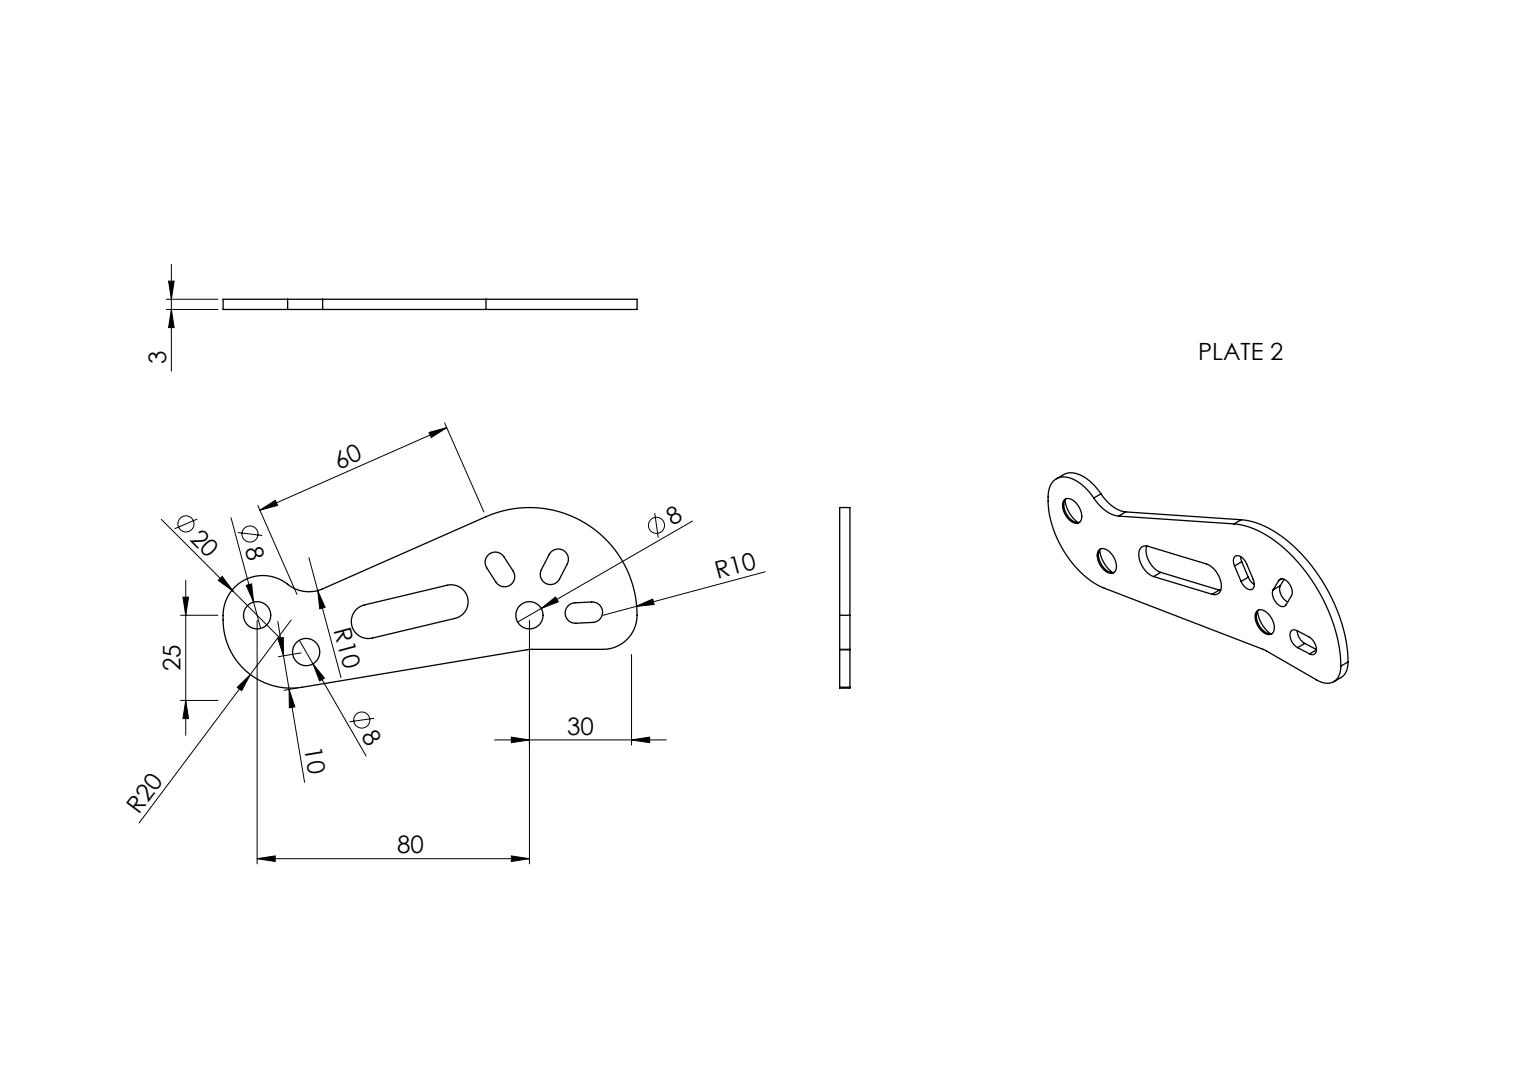
ISO-10303-21;
HEADER;
FILE_DESCRIPTION (('STEP AP214'),
    '1' );
FILE_NAME ('plate 2.step',
    '2026-10-31T03:41:51',
    ( '' ),
    ( '' ),
    'SwSTEP 2.0',
    'SolidWorks 2026',
    '' );
FILE_SCHEMA (( 'AUTOMOTIVE_DESIGN' ));
ENDSEC;

DATA;
#18=ORIENTED_EDGE ( 'NONE', *, *, #2231, .T. ) ;
#36=ORIENTED_EDGE ( 'NONE', *, *, #1393, .T. ) ;
#45=FACE_OUTER_BOUND ( 'NONE', #11478, .T. ) ;
#51=CARTESIAN_POINT ( 'NONE',  ( 69.97572749000833880, 15.55805301486455683, 6.000000000000000000 ) ) ;
#52=ORIENTED_EDGE ( 'NONE', *, *, #8148, .F. ) ;
#97=ADVANCED_FACE ( 'NONE', ( #2039 ), #6726, .F. ) ;
#108=VERTEX_POINT ( 'NONE', #10337 ) ;
#117=CARTESIAN_POINT ( 'NONE',  ( 76.00000000000000000, 4.898587196589422689E-16, 6.000000000000000000 ) ) ;
#123=EDGE_LOOP ( 'NONE', ( #11142, #6694, #3229, #3331, #1477 ) ) ;
#135=CARTESIAN_POINT ( 'NONE',  ( 80.00000000000000000, 0.000000000000000000, 5.500000000000000000 ) ) ;
#145=VECTOR ( 'NONE', #5198, 1000.000000000000000 ) ;
#158=DIRECTION ( 'NONE',  ( 1.000000000000000000, 0.000000000000000000, 0.000000000000000000 ) ) ;
#160=VECTOR ( 'NONE', #9182, 1000.000000000000000 ) ;
#161=LINE ( 'NONE', #4805, #11382 ) ;
#186=PLANE ( 'NONE',  #13689 ) ;
#193=ORIENTED_EDGE ( 'NONE', *, *, #9161, .T. ) ;
#211=EDGE_CURVE ( 'NONE', #12769, #12700, #14657, .T. ) ;
#214=VERTEX_POINT ( 'NONE', #2422 ) ;
#216=CARTESIAN_POINT ( 'NONE',  ( 80.00000000000000000, 0.000000000000000000, -131.1575142076926852 ) ) ;
#224=DIRECTION ( 'NONE',  ( -0.000000000000000000, -0.000000000000000000, -1.000000000000000000 ) ) ;
#233=DIRECTION ( 'NONE',  ( 1.000000000000000000, 0.000000000000000000, 0.000000000000000000 ) ) ;
#234=ADVANCED_FACE ( 'NONE', ( #9266 ), #13953, .F. ) ;
#239=DIRECTION ( 'NONE',  ( 0.9728364810787194505, 0.2314933715733012709, -0.000000000000000000 ) ) ;
#243=CARTESIAN_POINT ( 'NONE',  ( 31.51081190520435626, 3.030430839836910639, 2.999999999999999112 ) ) ;
#244=LINE ( 'NONE', #4960, #10717 ) ;
#246=CARTESIAN_POINT ( 'NONE',  ( 10.40394475573011945, -10.79473832354794460, 6.000000000000000000 ) ) ;
#247=ORIENTED_EDGE ( 'NONE', *, *, #4486, .T. ) ;
#250=CARTESIAN_POINT ( 'NONE',  ( -5.999999999999999112, 0.000000000000000000, 3.000000000000000000 ) ) ;
#253=( LENGTH_UNIT ( ) NAMED_UNIT ( * ) SI_UNIT ( .MILLI., .METRE. ) );
#264=EDGE_CURVE ( 'NONE', #12037, #12700, #1561, .T. ) ;
#289=DIRECTION ( 'NONE',  ( 1.000000000000000000, 0.000000000000000000, -0.000000000000000000 ) ) ;
#310=FACE_OUTER_BOUND ( 'NONE', #10572, .T. ) ;
#314=DIRECTION ( 'NONE',  ( -0.000000000000000000, -0.000000000000000000, -1.000000000000000000 ) ) ;
#326=DIRECTION ( 'NONE',  ( 0.000000000000000000, 0.000000000000000000, 1.000000000000000000 ) ) ;
#332=DIRECTION ( 'NONE',  ( 1.000000000000000000, 0.000000000000000000, 0.000000000000000000 ) ) ;
#340=EDGE_CURVE ( 'NONE', #7818, #11509, #2563, .T. ) ;
#344=EDGE_CURVE ( 'NONE', #1013, #13731, #244, .T. ) ;
#351=DIRECTION ( 'NONE',  ( -0.000000000000000000, -0.000000000000000000, -1.000000000000000000 ) ) ;
#372=DIRECTION ( 'NONE',  ( -0.000000000000000000, -0.000000000000000000, 1.000000000000000000 ) ) ;
#401=AXIS2_PLACEMENT_3D ( 'NONE', #216, #3759, #10608 ) ;
#412=LINE ( 'NONE', #6346, #4643 ) ;
#413=DIRECTION ( 'NONE',  ( -0.000000000000000000, -0.000000000000000000, 1.000000000000000000 ) ) ;
#445=CARTESIAN_POINT ( 'NONE',  ( 19.25177984293775424, 7.759396820770413150, 6.000000000000005329 ) ) ;
#454=DIRECTION ( 'NONE',  ( -1.000000000000000000, 0.000000000000000000, 0.000000000000000000 ) ) ;
#460=EDGE_CURVE ( 'NONE', #5313, #7859, #6354, .T. ) ;
#466=ORIENTED_EDGE ( 'NONE', *, *, #12652, .F. ) ;
#470=ORIENTED_EDGE ( 'NONE', *, *, #13886, .T. ) ;
#480=CARTESIAN_POINT ( 'NONE',  ( -9.999999999999998224, 0.000000000000000000, -131.1575142076926852 ) ) ;
#481=ORIENTED_EDGE ( 'NONE', *, *, #1964, .T. ) ;
#487=CYLINDRICAL_SURFACE ( 'NONE', #11244, 5.999999999999999112 ) ;
#491=CARTESIAN_POINT ( 'NONE',  ( 67.23404255319148604, 28.93147646537027384, -131.1575142076926852 ) ) ;
#501=DIRECTION ( 'NONE',  ( -1.000000000000000000, 0.000000000000000000, 0.000000000000000000 ) ) ;
#511=EDGE_CURVE ( 'NONE', #12603, #7404, #14471, .T. ) ;
#518=CARTESIAN_POINT ( 'NONE',  ( 80.00000000000000000, 0.000000000000000000, -131.1575142076926852 ) ) ;
#534=VECTOR ( 'NONE', #1828, 1000.000000000000000 ) ;
#538=CARTESIAN_POINT ( 'NONE',  ( 69.97572749000833880, 15.55805301486455683, 2.999999999999999112 ) ) ;
#541=ORIENTED_EDGE ( 'NONE', *, *, #8159, .F. ) ;
#548=LINE ( 'NONE', #11154, #9933 ) ;
#550=LINE ( 'NONE', #5266, #14058 ) ;
#554=CARTESIAN_POINT ( 'NONE',  ( 31.51081190520435626, 3.030430839836910639, 2.999999999999999112 ) ) ;
#555=VERTEX_POINT ( 'NONE', #13184 ) ;
#558=FILL_AREA_STYLE ('',( #14571 ) ) ;
#562=ORIENTED_EDGE ( 'NONE', *, *, #11530, .T. ) ;
#578=VECTOR ( 'NONE', #11844, 1000.000000000000000 ) ;
#596=ORIENTED_EDGE ( 'NONE', *, *, #3350, .T. ) ;
#605=VECTOR ( 'NONE', #5620, 1000.000000000000114 ) ;
#614=AXIS2_PLACEMENT_3D ( 'NONE', #11477, #5656, #729 ) ;
#664=DIRECTION ( 'NONE',  ( 0.000000000000000000, 0.000000000000000000, 1.000000000000000000 ) ) ;
#666=PRODUCT_CONTEXT ( 'NONE', #2624, 'mechanical' ) ;
#677=VERTEX_POINT ( 'NONE', #4761 ) ;
#679=DIRECTION ( 'NONE',  ( 1.000000000000000000, 0.000000000000000000, 0.000000000000000000 ) ) ;
#682=ORIENTED_EDGE ( 'NONE', *, *, #8049, .T. ) ;
#708=AXIS2_PLACEMENT_3D ( 'NONE', #5305, #9976, #14676 ) ;
#714=LINE ( 'NONE', #863, #6086 ) ;
#729=DIRECTION ( 'NONE',  ( 1.000000000000000000, 0.000000000000000000, 0.000000000000000000 ) ) ;
#746=ADVANCED_FACE ( 'NONE', ( #2228 ), #6914, .F. ) ;
#747=CARTESIAN_POINT ( 'NONE',  ( -4.000000000000000000, 0.000000000000000000, 6.000000000000000000 ) ) ;
#779=EDGE_CURVE ( 'NONE', #11305, #1805, #11744, .T. ) ;
#788=ORIENTED_EDGE ( 'NONE', *, *, #5470, .F. ) ;
#794=AXIS2_PLACEMENT_3D ( 'NONE', #9301, #8135, #991 ) ;
#854=AXIS2_PLACEMENT_3D ( 'NONE', #10836, #10689, #6078 ) ;
#855=AXIS2_PLACEMENT_3D ( 'NONE', #5788, #13776, #8092 ) ;
#861=DIRECTION ( 'NONE',  ( 0.000000000000000000, 0.000000000000000000, 1.000000000000000000 ) ) ;
#862=FACE_OUTER_BOUND ( 'NONE', #14868, .T. ) ;
#863=CARTESIAN_POINT ( 'NONE',  ( 31.51081190520435626, 3.030430839836910639, 2.999999999999999112 ) ) ;
#864=AXIS2_PLACEMENT_3D ( 'NONE', #2501, #3652, #7037 ) ;
#870=ORIENTED_EDGE ( 'NONE', *, *, #10742, .T. ) ;
#877=ORIENTED_EDGE ( 'NONE', *, *, #7016, .T. ) ;
#878=CARTESIAN_POINT ( 'NONE',  ( -9.999999999999998224, 0.000000000000000000, -131.1575142076926852 ) ) ;
#904=EDGE_LOOP ( 'NONE', ( #11080, #1437, #4193, #4487 ) ) ;
#913=LINE ( 'NONE', #4463, #605 ) ;
#926=AXIS2_PLACEMENT_3D ( 'NONE', #8242, #7946, #12629 ) ;
#937=CIRCLE ( 'NONE', #9527, 4.000000000000003553 ) ;
#961=( LENGTH_UNIT ( ) NAMED_UNIT ( * ) SI_UNIT ( .MILLI., .METRE. ) );
#976=DIRECTION ( 'NONE',  ( -1.000000000000000000, 0.000000000000000000, 0.000000000000000000 ) ) ;
#977=VECTOR ( 'NONE', #5224, 1000.000000000000000 ) ;
#979=ORIENTED_EDGE ( 'NONE', *, *, #5847, .F. ) ;
#981=CARTESIAN_POINT ( 'NONE',  ( 15.21482963846748504, 16.90833299098317610, 3.000000000000002665 ) ) ;
#991=DIRECTION ( 'NONE',  ( -1.000000000000000000, 0.000000000000000000, -0.000000000000000000 ) ) ;
#994=DIRECTION ( 'NONE',  ( 1.000000000000000000, 0.000000000000000000, 0.000000000000000000 ) ) ;
#1013=VERTEX_POINT ( 'NONE', #13943 ) ;
#1041=ORIENTED_EDGE ( 'NONE', *, *, #264, .T. ) ;
#1044=EDGE_CURVE ( 'NONE', #5009, #9526, #161, .T. ) ;
#1059=DIRECTION ( 'NONE',  ( -0.000000000000000000, -0.000000000000000000, 1.000000000000000000 ) ) ;
#1075=EDGE_LOOP ( 'NONE', ( #12142, #6161 ) ) ;
#1078=ORIENTED_EDGE ( 'NONE', *, *, #5790, .F. ) ;
#1079=EDGE_LOOP ( 'NONE', ( #2513, #15023, #6182, #877 ) ) ;
#1098=ORIENTED_EDGE ( 'NONE', *, *, #9625, .T. ) ;
#1109=LINE ( 'NONE', #4729, #8437 ) ;
#1114=CIRCLE ( 'NONE', #5058, 2.999999999999975131 ) ;
#1136=VERTEX_POINT ( 'NONE', #10785 ) ;
#1161=PLANE ( 'NONE',  #7041 ) ;
#1163=( GEOMETRIC_REPRESENTATION_CONTEXT ( 3 ) GLOBAL_UNCERTAINTY_ASSIGNED_CONTEXT ( ( #8003 ) ) GLOBAL_UNIT_ASSIGNED_CONTEXT ( ( #961, #13644, #10039 ) ) REPRESENTATION_CONTEXT ( 'NONE', 'WORKASPACE' ) );
#1174=CARTESIAN_POINT ( 'NONE',  ( 8.961831343790189308, 9.104486995144789319, 3.000000000000002665 ) ) ;
#1185=CARTESIAN_POINT ( 'NONE',  ( 83.50748565343083385, 13.38500995229612478, 2.999999999999999112 ) ) ;
#1218=DIRECTION ( 'NONE',  ( 0.000000000000000000, 0.000000000000000000, -1.000000000000000000 ) ) ;
#1225=DIRECTION ( 'NONE',  ( 0.2314933715733012709, -0.9728364810787194505, 0.000000000000000000 ) ) ;
#1236=CYLINDRICAL_SURFACE ( 'NONE', #401, 31.62277660168379256 ) ;
#1247=EDGE_CURVE ( 'NONE', #7097, #4081, #548, .T. ) ;
#1250=CARTESIAN_POINT ( 'NONE',  ( 10.40394475573011945, -10.79473832354794460, 6.000000000000000000 ) ) ;
#1253=LINE ( 'NONE', #10562, #4367 ) ;
#1280=LINE ( 'NONE', #8132, #6582 ) ;
#1287=ORIENTED_EDGE ( 'NONE', *, *, #1044, .T. ) ;
#1297=ORIENTED_EDGE ( 'NONE', *, *, #12952, .T. ) ;
#1300=FACE_OUTER_BOUND ( 'NONE', #5332, .T. ) ;
#1346=CARTESIAN_POINT ( 'NONE',  ( 18.40394475573011945, -10.79473832354794460, 6.000000000000000000 ) ) ;
#1361=LINE ( 'NONE', #2683, #9152 ) ;
#1364=ORIENTED_EDGE ( 'NONE', *, *, #11141, .T. ) ;
#1369=CARTESIAN_POINT ( 'NONE',  ( 0.000000000000000000, 0.000000000000000000, 5.500000000000000000 ) ) ;
#1376=AXIS2_PLACEMENT_3D ( 'NONE', #7353, #6187, #9640 ) ;
#1382=DIRECTION ( 'NONE',  ( -0.000000000000000000, -0.000000000000000000, 1.000000000000000000 ) ) ;
#1384=EDGE_CURVE ( 'NONE', #1805, #14461, #7483, .T. ) ;
#1392=AXIS2_PLACEMENT_3D ( 'NONE', #12930, #7026, #11705 ) ;
#1393=EDGE_CURVE ( 'NONE', #11633, #7557, #3313, .T. ) ;
#1407=ADVANCED_FACE ( 'NONE', ( #862 ), #10161, .F. ) ;
#1411=CARTESIAN_POINT ( 'NONE',  ( 80.00000000000000000, 0.000000000000000000, 3.000000000000002665 ) ) ;
#1419=AXIS2_PLACEMENT_3D ( 'NONE', #9521, #10244, #11889 ) ;
#1425=LINE ( 'NONE', #5277, #6096 ) ;
#1429=AXIS2_PLACEMENT_3D ( 'NONE', #14450, #12280, #8594 ) ;
#1437=ORIENTED_EDGE ( 'NONE', *, *, #3878, .F. ) ;
#1453=CARTESIAN_POINT ( 'NONE',  ( 74.00000000000000000, 0.000000000000000000, 5.500000000000000000 ) ) ;
#1469=CARTESIAN_POINT ( 'NONE',  ( 80.00000000000000000, -9.999999999999994671, -131.1575142076926852 ) ) ;
#1470=DIRECTION ( 'NONE',  ( 0.000000000000000000, 0.000000000000000000, -1.000000000000000000 ) ) ;
#1477=ORIENTED_EDGE ( 'NONE', *, *, #1540, .F. ) ;
#1482=VERTEX_POINT ( 'NONE', #8309 ) ;
#1494=ORIENTED_EDGE ( 'NONE', *, *, #4486, .F. ) ;
#1502=DIRECTION ( 'NONE',  ( 0.000000000000000000, 0.000000000000000000, 1.000000000000000000 ) ) ;
#1518=DIRECTION ( 'NONE',  ( -0.000000000000000000, -0.000000000000000000, 1.000000000000000000 ) ) ;
#1523=DIRECTION ( 'NONE',  ( 1.000000000000000000, 0.000000000000000000, 0.000000000000000000 ) ) ;
#1524=VECTOR ( 'NONE', #2212, 1000.000000000000000 ) ;
#1526=DIRECTION ( 'NONE',  ( 0.000000000000000000, 0.000000000000000000, 1.000000000000000000 ) ) ;
#1527=EDGE_CURVE ( 'NONE', #14446, #9599, #1641, .T. ) ;
#1532=EDGE_LOOP ( 'NONE', ( #3117, #4460, #13209, #9461, #14696 ) ) ;
#1539=CARTESIAN_POINT ( 'NONE',  ( 10.00000000000000178, -1.390791565672601315, 3.000000000000002665 ) ) ;
#1540=EDGE_CURVE ( 'NONE', #14414, #5535, #6005, .T. ) ;
#1551=EDGE_LOOP ( 'NONE', ( #3528, #541, #2755, #9080, #10467 ) ) ;
#1559=ORIENTED_EDGE ( 'NONE', *, *, #5818, .T. ) ;
#1560=DIRECTION ( 'NONE',  ( 1.000000000000000000, 0.000000000000000000, 0.000000000000000000 ) ) ;
#1561=LINE ( 'NONE', #480, #145 ) ;
#1570=EDGE_CURVE ( 'NONE', #2216, #4678, #12832, .T. ) ;
#1571=EDGE_CURVE ( 'NONE', #13989, #10279, #3470, .T. ) ;
#1589=VECTOR ( 'NONE', #7529, 1000.000000000000000 ) ;
#1603=EDGE_CURVE ( 'NONE', #1860, #1482, #7085, .T. ) ;
#1641=CIRCLE ( 'NONE', #6308, 4.999999999999997335 ) ;
#1643=DIRECTION ( 'NONE',  ( 0.04874958797097354163, -0.9988110320138942066, 0.000000000000000000 ) ) ;
#1655=( NAMED_UNIT ( * ) SI_UNIT ( $, .STERADIAN. ) SOLID_ANGLE_UNIT ( ) );
#1659=ORIENTED_EDGE ( 'NONE', *, *, #4604, .F. ) ;
#1669=ORIENTED_EDGE ( 'NONE', *, *, #460, .T. ) ;
#1671=VECTOR ( 'NONE', #11024, 1000.000000000000000 ) ;
#1675=VECTOR ( 'NONE', #9164, 1000.000000000000227 ) ;
#1682=ORIENTED_EDGE ( 'NONE', *, *, #11497, .T. ) ;
#1685=CARTESIAN_POINT ( 'NONE',  ( 85.79342132543153809, 17.83186255874426962, 6.000000000000000000 ) ) ;
#1693=ORIENTED_EDGE ( 'NONE', *, *, #9686, .T. ) ;
#1703=LINE ( 'NONE', #8538, #10944 ) ;
#1704=DIRECTION ( 'NONE',  ( 1.000000000000000000, 0.000000000000000000, 0.000000000000000000 ) ) ;
#1706=ORIENTED_EDGE ( 'NONE', *, *, #3827, .F. ) ;
#1719=VECTOR ( 'NONE', #8136, 1000.000000000000000 ) ;
#1725=CARTESIAN_POINT ( 'NONE',  ( 56.98919079003883326, 3.953582723775848962, 2.999999999999999112 ) ) ;
#1732=EDGE_CURVE ( 'NONE', #3235, #9526, #15133, .T. ) ;
#1734=EDGE_CURVE ( 'NONE', #14461, #2630, #1703, .T. ) ;
#1769=EDGE_CURVE ( 'NONE', #13658, #11133, #8990, .T. ) ;
#1776=CIRCLE ( 'NONE', #6200, 5.999999999999999112 ) ;
#1788=EDGE_LOOP ( 'NONE', ( #2878, #682, #5226, #13096 ) ) ;
#1800=CARTESIAN_POINT ( 'NONE',  ( -9.999999999999992895, -25.00000000000000000, -131.1575142076926852 ) ) ;
#1803=DIRECTION ( 'NONE',  ( 0.000000000000000000, 0.000000000000000000, 1.000000000000000000 ) ) ;
#1805=VERTEX_POINT ( 'NONE', #5475 ) ;
#1808=ORIENTED_EDGE ( 'NONE', *, *, #6015, .T. ) ;
#1828=DIRECTION ( 'NONE',  ( -0.000000000000000000, -0.000000000000000000, -1.000000000000000000 ) ) ;
#1830=DIRECTION ( 'NONE',  ( 1.000000000000000000, 0.000000000000000000, 0.000000000000000000 ) ) ;
#1860=VERTEX_POINT ( 'NONE', #11521 ) ;
#1865=CYLINDRICAL_SURFACE ( 'NONE', #10935, 2.999999999999988898 ) ;
#1874=AXIS2_PLACEMENT_3D ( 'NONE', #1369, #10753, #11665 ) ;
#1895=CARTESIAN_POINT ( 'NONE',  ( 76.00000000000000000, 4.898587196589422689E-16, 5.500000000000005329 ) ) ;
#1905=CARTESIAN_POINT ( 'NONE',  ( 0.000000000000000000, 0.000000000000000000, 5.500000000000000000 ) ) ;
#1913=ORIENTED_EDGE ( 'NONE', *, *, #9541, .F. ) ;
#1915=STYLED_ITEM ( 'NONE', ( #6714 ), #15172 ) ;
#1921=AXIS2_PLACEMENT_3D ( 'NONE', #4330, #13703, #3182 ) ;
#1925=DIRECTION ( 'NONE',  ( 0.000000000000000000, 0.000000000000000000, 1.000000000000000000 ) ) ;
#1929=DIRECTION ( 'NONE',  ( -1.000000000000000000, 0.000000000000000000, 0.000000000000000000 ) ) ;
#1946=AXIS2_PLACEMENT_3D ( 'NONE', #3215, #10121, #11276 ) ;
#1947=CARTESIAN_POINT ( 'NONE',  ( 70.16198417812034904, 9.730076655429538590, 2.999999999999999112 ) ) ;
#1964=EDGE_CURVE ( 'NONE', #4081, #10279, #8485, .T. ) ;
#1976=ORIENTED_EDGE ( 'NONE', *, *, #6296, .T. ) ;
#1981=ADVANCED_FACE ( 'NONE', ( #5985 ), #3522, .F. ) ;
#1992=ADVANCED_FACE ( 'NONE', ( #8139 ), #6987, .F. ) ;
#2001=CARTESIAN_POINT ( 'NONE',  ( 101.6227766016837819, 5.204170427930421283E-15, -131.1575142076926852 ) ) ;
#2020=LINE ( 'NONE', #13546, #4525 ) ;
#2029=SURFACE_STYLE_FILL_AREA ( #558 ) ;
#2033=DIRECTION ( 'NONE',  ( 1.000000000000000000, 0.000000000000000000, 0.000000000000000000 ) ) ;
#2039=FACE_OUTER_BOUND ( 'NONE', #8512, .T. ) ;
#2044=DIRECTION ( 'NONE',  ( -0.000000000000000000, -0.000000000000000000, 1.000000000000000000 ) ) ;
#2060=DIRECTION ( 'NONE',  ( 0.000000000000000000, 0.000000000000000000, 1.000000000000000000 ) ) ;
#2062=ORIENTED_EDGE ( 'NONE', *, *, #1527, .F. ) ;
#2086=FACE_OUTER_BOUND ( 'NONE', #13410, .T. ) ;
#2109=CARTESIAN_POINT ( 'NONE',  ( 0.000000000000000000, 0.000000000000000000, 3.000000000000000000 ) ) ;
#2112=CARTESIAN_POINT ( 'NONE',  ( 83.50748565343083385, 13.38500995229612478, 2.999999999999999112 ) ) ;
#2117=ORIENTED_EDGE ( 'NONE', *, *, #1247, .F. ) ;
#2133=DIRECTION ( 'NONE',  ( -0.000000000000000000, -0.000000000000000000, 1.000000000000000000 ) ) ;
#2137=DIRECTION ( 'NONE',  ( 0.000000000000000000, 0.000000000000000000, 1.000000000000000000 ) ) ;
#2151=VECTOR ( 'NONE', #14804, 1000.000000000000000 ) ;
#2161=CIRCLE ( 'NONE', #7069, 4.000000000000000000 ) ;
#2187=ORIENTED_EDGE ( 'NONE', *, *, #2481, .T. ) ;
#2190=AXIS2_PLACEMENT_3D ( 'NONE', #15212, #11795, #5966 ) ;
#2191=AXIS2_PLACEMENT_3D ( 'NONE', #1905, #6598, #10277 ) ;
#2193=DIRECTION ( 'NONE',  ( 2.081668171172168513E-16, -1.000000000000000000, 0.000000000000000000 ) ) ;
#2212=DIRECTION ( 'NONE',  ( -0.000000000000000000, -0.000000000000000000, -1.000000000000000000 ) ) ;
#2216=VERTEX_POINT ( 'NONE', #5606 ) ;
#2225=CARTESIAN_POINT ( 'NONE',  ( 75.20570977803312473, 12.97982004111159959, 2.999999999999999112 ) ) ;
#2228=FACE_OUTER_BOUND ( 'NONE', #904, .T. ) ;
#2231=EDGE_CURVE ( 'NONE', #9019, #14061, #10282, .T. ) ;
#2281=DIRECTION ( 'NONE',  ( -0.000000000000000000, -0.000000000000000000, -1.000000000000000000 ) ) ;
#2286=ORIENTED_EDGE ( 'NONE', *, *, #14935, .F. ) ;
#2287=EDGE_CURVE ( 'NONE', #2216, #1136, #10843, .T. ) ;
#2288=DIRECTION ( 'NONE',  ( 1.000000000000000000, 0.000000000000000000, 0.000000000000000000 ) ) ;
#2290=DIRECTION ( 'NONE',  ( -1.000000000000000000, 0.000000000000000000, 0.000000000000000000 ) ) ;
#2314=ORIENTED_EDGE ( 'NONE', *, *, #3325, .F. ) ;
#2320=CIRCLE ( 'NONE', #10417, 20.00000000000000000 ) ;
#2329=EDGE_CURVE ( 'NONE', #1136, #13200, #12726, .T. ) ;
#2330=ORIENTED_EDGE ( 'NONE', *, *, #10701, .F. ) ;
#2339=DIRECTION ( 'NONE',  ( -0.000000000000000000, -0.000000000000000000, -1.000000000000000000 ) ) ;
#2341=ORIENTED_EDGE ( 'NONE', *, *, #7033, .F. ) ;
#2356=CARTESIAN_POINT ( 'NONE',  ( 20.40394475573011590, -10.79473832354794460, 22.47056274847713908 ) ) ;
#2410=DIRECTION ( 'NONE',  ( 1.000000000000000000, 0.000000000000000000, 0.000000000000000000 ) ) ;
#2416=CARTESIAN_POINT ( 'NONE',  ( 74.00000000000000000, 0.000000000000000000, 3.000000000000000000 ) ) ;
#2419=ORIENTED_EDGE ( 'NONE', *, *, #8213, .T. ) ;
#2422=CARTESIAN_POINT ( 'NONE',  ( 84.00000000000000000, 0.000000000000000000, 5.500000000000005329 ) ) ;
#2429=EDGE_CURVE ( 'NONE', #7404, #12603, #10351, .T. ) ;
#2441=VERTEX_POINT ( 'NONE', #12795 ) ;
#2458=VECTOR ( 'NONE', #3595, 1000.000000000000000 ) ;
#2467=ORIENTED_EDGE ( 'NONE', *, *, #12952, .F. ) ;
#2470=DIRECTION ( 'NONE',  ( -1.000000000000000000, 0.000000000000000000, 0.000000000000000000 ) ) ;
#2481=EDGE_CURVE ( 'NONE', #7818, #1860, #5212, .T. ) ;
#2485=CARTESIAN_POINT ( 'NONE',  ( 88.46153288930041469, 16.46030115554384565, 2.999999999999999112 ) ) ;
#2501=CARTESIAN_POINT ( 'NONE',  ( 98.48580539929344013, 0.9022481406819604643, 2.999999999999999112 ) ) ;
#2513=ORIENTED_EDGE ( 'NONE', *, *, #10110, .F. ) ;
#2522=AXIS2_PLACEMENT_3D ( 'NONE', #3024, #11541, #8010 ) ;
#2536=FACE_OUTER_BOUND ( 'NONE', #4180, .T. ) ;
#2555=DIRECTION ( 'NONE',  ( -1.000000000000000000, 0.000000000000000000, 0.000000000000000000 ) ) ;
#2563=LINE ( 'NONE', #11928, #3125 ) ;
#2568=CYLINDRICAL_SURFACE ( 'NONE', #9771, 6.000000000000005329 ) ;
#2578=ORIENTED_EDGE ( 'NONE', *, *, #3073, .T. ) ;
#2588=SHAPE_REPRESENTATION ( 'plate 2', ( #1376 ), #5367 ) ;
#2600=CARTESIAN_POINT ( 'NONE',  ( 72.49759028996474797, 17.18292470770558822, 3.000000000000000000 ) ) ;
#2602=EDGE_LOOP ( 'NONE', ( #9382, #1287, #4247, #1078 ) ) ;
#2621=EDGE_CURVE ( 'NONE', #11509, #677, #4484, .T. ) ;
#2624=APPLICATION_CONTEXT ( 'automotive_design' ) ;
#2630=VERTEX_POINT ( 'NONE', #4272 ) ;
#2641=ORIENTED_EDGE ( 'NONE', *, *, #8239, .T. ) ;
#2660=DIRECTION ( 'NONE',  ( 0.000000000000000000, 0.000000000000000000, 1.000000000000000000 ) ) ;
#2662=DIRECTION ( 'NONE',  ( -1.000000000000000000, 0.000000000000000000, 0.000000000000000000 ) ) ;
#2672=ORIENTED_EDGE ( 'NONE', *, *, #6777, .F. ) ;
#2678=DIRECTION ( 'NONE',  ( 1.000000000000000000, 0.000000000000000000, 0.000000000000000000 ) ) ;
#2680=LINE ( 'NONE', #13423, #8264 ) ;
#2683=CARTESIAN_POINT ( 'NONE',  ( 98.33955663538051795, 3.898681236723621879, 2.999999999999999112 ) ) ;
#2701=AXIS2_PLACEMENT_3D ( 'NONE', #14538, #8610, #9772 ) ;
#2706=DIRECTION ( 'NONE',  ( 1.000000000000000000, 0.000000000000000000, 0.000000000000000000 ) ) ;
#2713=EDGE_LOOP ( 'NONE', ( #8843, #12332, #6690, #8767, #1297 ) ) ;
#2720=FACE_OUTER_BOUND ( 'NONE', #3492, .T. ) ;
#2721=EDGE_CURVE ( 'NONE', #14061, #6410, #1776, .T. ) ;
#2728=ORIENTED_EDGE ( 'NONE', *, *, #1769, .F. ) ;
#2752=ORIENTED_EDGE ( 'NONE', *, *, #8228, .F. ) ;
#2755=ORIENTED_EDGE ( 'NONE', *, *, #6452, .F. ) ;
#2784=EDGE_CURVE ( 'NONE', #214, #4354, #1109, .T. ) ;
#2793=CARTESIAN_POINT ( 'NONE',  ( 91.12964445316929130, 15.08873975234342701, 2.999999999999999112 ) ) ;
#2811=EDGE_CURVE ( 'NONE', #7859, #7552, #11625, .T. ) ;
#2849=DIRECTION ( 'NONE',  ( 0.000000000000000000, 0.000000000000000000, 1.000000000000000000 ) ) ;
#2855=DIRECTION ( 'NONE',  ( 0.000000000000000000, 0.000000000000000000, 1.000000000000000000 ) ) ;
#2856=ADVANCED_FACE ( 'NONE', ( #15106 ), #4500, .T. ) ;
#2877=ORIENTED_EDGE ( 'NONE', *, *, #4223, .T. ) ;
#2878=ORIENTED_EDGE ( 'NONE', *, *, #6158, .T. ) ;
#2879=CYLINDRICAL_SURFACE ( 'NONE', #9523, 2.999999999999988898 ) ;
#2895=VERTEX_POINT ( 'NONE', #2416 ) ;
#2903=VECTOR ( 'NONE', #3984, 1000.000000000000000 ) ;
#2904=DIRECTION ( 'NONE',  ( -0.000000000000000000, -0.000000000000000000, 1.000000000000000000 ) ) ;
#2908=LINE ( 'NONE', #11048, #977 ) ;
#2915=EDGE_CURVE ( 'NONE', #13200, #4678, #7219, .T. ) ;
#2928=LINE ( 'NONE', #9607, #7239 ) ;
#2932=AXIS2_PLACEMENT_3D ( 'NONE', #1185, #13241, #3781 ) ;
#2952=ORIENTED_EDGE ( 'NONE', *, *, #6015, .F. ) ;
#2959=DIRECTION ( 'NONE',  ( -1.000000000000000000, 0.000000000000000000, 0.000000000000000000 ) ) ;
#2960=FACE_BOUND ( 'NONE', #10830, .T. ) ;
#2970=EDGE_CURVE ( 'NONE', #2441, #9761, #14339, .T. ) ;
#2982=FACE_OUTER_BOUND ( 'NONE', #3019, .T. ) ;
#2986=CARTESIAN_POINT ( 'NONE',  ( 80.00000000000000000, -9.999999999999994671, 3.000000000000002665 ) ) ;
#2987=ORIENTED_EDGE ( 'NONE', *, *, #2970, .T. ) ;
#2991=VERTEX_POINT ( 'NONE', #11137 ) ;
#3003=DIRECTION ( 'NONE',  ( -1.000000000000000000, 0.000000000000000000, 0.000000000000000000 ) ) ;
#3012=ORIENTED_EDGE ( 'NONE', *, *, #7407, .F. ) ;
#3019=EDGE_LOOP ( 'NONE', ( #3012, #7526, #11091, #2728 ) ) ;
#3023=CARTESIAN_POINT ( 'NONE',  ( 32.66827876307085887, -1.833751565556681173, 2.999999999999999112 ) ) ;
#3024=CARTESIAN_POINT ( 'NONE',  ( 98.48580539929344013, 0.9022481406819604643, 6.000000000000000000 ) ) ;
#3073=EDGE_CURVE ( 'NONE', #555, #6387, #3306, .T. ) ;
#3074=CARTESIAN_POINT ( 'NONE',  ( 101.4858053992934401, 0.9022481406819604643, 6.000000000000000000 ) ) ;
#3079=AXIS2_PLACEMENT_3D ( 'NONE', #11309, #10083, #12306 ) ;
#3091=ORIENTED_EDGE ( 'NONE', *, *, #344, .T. ) ;
#3092=ORIENTED_EDGE ( 'NONE', *, *, #1734, .T. ) ;
#3093=ORIENTED_EDGE ( 'NONE', *, *, #211, .F. ) ;
#3098=CARTESIAN_POINT ( 'NONE',  ( 58.14665764790533586, -0.9105996816177489572, 6.000000000000000000 ) ) ;
#3109=AXIS2_PLACEMENT_3D ( 'NONE', #10354, #2137, #13747 ) ;
#3117=ORIENTED_EDGE ( 'NONE', *, *, #3440, .F. ) ;
#3125=VECTOR ( 'NONE', #6109, 1000.000000000000227 ) ;
#3158=CYLINDRICAL_SURFACE ( 'NONE', #6590, 9.999999999999994671 ) ;
#3168=DIRECTION ( 'NONE',  ( -0.9148936170212765839, -0.4036950204470271530, 0.000000000000000000 ) ) ;
#3180=ORIENTED_EDGE ( 'NONE', *, *, #6159, .F. ) ;
#3182=DIRECTION ( 'NONE',  ( 1.000000000000000000, 0.000000000000000000, 0.000000000000000000 ) ) ;
#3208=AXIS2_PLACEMENT_3D ( 'NONE', #9497, #10509, #14191 ) ;
#3215=CARTESIAN_POINT ( 'NONE',  ( 88.46153288930041469, 16.46030115554384565, 6.000000000000000000 ) ) ;
#3229=ORIENTED_EDGE ( 'NONE', *, *, #12328, .F. ) ;
#3235=VERTEX_POINT ( 'NONE', #7146 ) ;
#3258=ORIENTED_EDGE ( 'NONE', *, *, #1540, .T. ) ;
#3260=VECTOR ( 'NONE', #11218, 1000.000000000000000 ) ;
#3263=FACE_OUTER_BOUND ( 'NONE', #7626, .T. ) ;
#3265=DIRECTION ( 'NONE',  ( 1.000000000000000000, 0.000000000000000000, 0.000000000000000000 ) ) ;
#3268=CARTESIAN_POINT ( 'NONE',  ( 70.16198417812034904, 9.730076655429538590, 2.999999999999999112 ) ) ;
#3295=ORIENTED_EDGE ( 'NONE', *, *, #8552, .T. ) ;
#3306=LINE ( 'NONE', #6768, #5754 ) ;
#3308=VERTEX_POINT ( 'NONE', #1685 ) ;
#3313=CIRCLE ( 'NONE', #12392, 4.000000000000000000 ) ;
#3319=ORIENTED_EDGE ( 'NONE', *, *, #8722, .T. ) ;
#3320=CARTESIAN_POINT ( 'NONE',  ( 88.46153288930041469, 16.46030115554384565, 2.999999999999999112 ) ) ;
#3325=EDGE_CURVE ( 'NONE', #9731, #15027, #14526, .T. ) ;
#3326=ORIENTED_EDGE ( 'NONE', *, *, #11310, .T. ) ;
#3329=EDGE_CURVE ( 'NONE', #9761, #6202, #5388, .T. ) ;
#3331=ORIENTED_EDGE ( 'NONE', *, *, #4868, .F. ) ;
#3333=AXIS2_PLACEMENT_3D ( 'NONE', #538, #2855, #10920 ) ;
#3350=EDGE_CURVE ( 'NONE', #9228, #555, #15090, .T. ) ;
#3351=DIRECTION ( 'NONE',  ( -0.000000000000000000, -0.000000000000000000, 1.000000000000000000 ) ) ;
#3354=CARTESIAN_POINT ( 'NONE',  ( 75.68384697807671557, 11.35494834827056110, 2.999999999999999112 ) ) ;
#3359=VERTEX_POINT ( 'NONE', #10974 ) ;
#3401=LINE ( 'NONE', #1947, #4671 ) ;
#3426=CIRCLE ( 'NONE', #4417, 6.000000000000005329 ) ;
#3435=DIRECTION ( 'NONE',  ( -1.000000000000000000, 0.000000000000000000, 0.000000000000000000 ) ) ;
#3440=EDGE_CURVE ( 'NONE', #8100, #1860, #9992, .T. ) ;
#3463=FACE_BOUND ( 'NONE', #14295, .T. ) ;
#3470=LINE ( 'NONE', #14072, #11202 ) ;
#3474=CARTESIAN_POINT ( 'NONE',  ( 8.961831343790189308, 9.104486995144789319, 6.000000000000000000 ) ) ;
#3492=EDGE_LOOP ( 'NONE', ( #9465, #3319, #12934, #6221 ) ) ;
#3522=CYLINDRICAL_SURFACE ( 'NONE', #1874, 5.999999999999999112 ) ;
#3528=ORIENTED_EDGE ( 'NONE', *, *, #9686, .F. ) ;
#3529=FACE_BOUND ( 'NONE', #5980, .T. ) ;
#3536=AXIS2_PLACEMENT_3D ( 'NONE', #10335, #4578, #9398 ) ;
#3559=DIRECTION ( 'NONE',  ( -0.9988110320138940956, -0.04874958797097371510, 0.000000000000000000 ) ) ;
#3562=CARTESIAN_POINT ( 'NONE',  ( 88.46153288930041469, 16.46030115554384565, 2.999999999999999112 ) ) ;
#3584=ORIENTED_EDGE ( 'NONE', *, *, #3697, .T. ) ;
#3595=DIRECTION ( 'NONE',  ( 0.000000000000000000, 0.000000000000000000, 1.000000000000000000 ) ) ;
#3610=FACE_OUTER_BOUND ( 'NONE', #14039, .T. ) ;
#3617=ORIENTED_EDGE ( 'NONE', *, *, #779, .T. ) ;
#3620=AXIS2_PLACEMENT_3D ( 'NONE', #6718, #6415, #11099 ) ;
#3622=CIRCLE ( 'NONE', #8783, 10.00000000000000000 ) ;
#3646=ORIENTED_EDGE ( 'NONE', *, *, #2231, .F. ) ;
#3652=DIRECTION ( 'NONE',  ( -0.000000000000000000, -0.000000000000000000, 1.000000000000000000 ) ) ;
#3676=DIRECTION ( 'NONE',  ( 0.9863939238321436376, 0.1643989873053573192, 0.000000000000000000 ) ) ;
#3684=ORIENTED_EDGE ( 'NONE', *, *, #5847, .T. ) ;
#3697=EDGE_CURVE ( 'NONE', #10279, #3235, #6197, .T. ) ;
#3702=DIRECTION ( 'NONE',  ( 0.000000000000000000, 0.000000000000000000, 1.000000000000000000 ) ) ;
#3714=DIRECTION ( 'NONE',  ( -0.000000000000000000, -0.000000000000000000, -1.000000000000000000 ) ) ;
#3718=ORIENTED_EDGE ( 'NONE', *, *, #12246, .T. ) ;
#3724=DIRECTION ( 'NONE',  ( 1.000000000000000000, 0.000000000000000000, 0.000000000000000000 ) ) ;
#3757=VERTEX_POINT ( 'NONE', #14345 ) ;
#3759=DIRECTION ( 'NONE',  ( 0.000000000000000000, 0.000000000000000000, 1.000000000000000000 ) ) ;
#3763=DIRECTION ( 'NONE',  ( -0.9988110320138940956, -0.04874958797097371510, -0.000000000000000000 ) ) ;
#3773=ORIENTED_EDGE ( 'NONE', *, *, #3325, .T. ) ;
#3781=DIRECTION ( 'NONE',  ( -0.4571871344001416926, -0.8893705212896291235, 0.000000000000000000 ) ) ;
#3810=CIRCLE ( 'NONE', #15113, 2.999999999999988898 ) ;
#3822=MANIFOLD_SOLID_BREP ( 'Cut-Extrude5', #9667 ) ;
#3823=EDGE_LOOP ( 'NONE', ( #52, #4946 ) ) ;
#3827=EDGE_CURVE ( 'NONE', #5429, #3757, #6658, .T. ) ;
#3838=VERTEX_POINT ( 'NONE', #1895 ) ;
#3873=( GEOMETRIC_REPRESENTATION_CONTEXT ( 3 ) GLOBAL_UNCERTAINTY_ASSIGNED_CONTEXT ( ( #5339 ) ) GLOBAL_UNIT_ASSIGNED_CONTEXT ( ( #10257, #9104, #5577 ) ) REPRESENTATION_CONTEXT ( 'NONE', 'WORKASPACE' ) );
#3878=EDGE_CURVE ( 'NONE', #14446, #5284, #7729, .T. ) ;
#3880=DIRECTION ( 'NONE',  ( 1.000000000000000000, 0.000000000000000000, 0.000000000000000000 ) ) ;
#3887=FACE_BOUND ( 'NONE', #11709, .T. ) ;
#3896=DIRECTION ( 'NONE',  ( 0.5416238976136762417, -0.8406209333187997235, 0.000000000000000000 ) ) ;
#3923=ORIENTED_EDGE ( 'NONE', *, *, #7892, .F. ) ;
#3937=VECTOR ( 'NONE', #9593, 1000.000000000000000 ) ;
#3947=FACE_OUTER_BOUND ( 'NONE', #9592, .T. ) ;
#3956=EDGE_LOOP ( 'NONE', ( #12824, #13348, #7937, #2117, #7805 ) ) ;
#3961=LINE ( 'NONE', #13171, #1671 ) ;
#3964=DIRECTION ( 'NONE',  ( -0.000000000000000000, -0.000000000000000000, 1.000000000000000000 ) ) ;
#3967=FACE_OUTER_BOUND ( 'NONE', #5270, .T. ) ;
#3976=ADVANCED_FACE ( 'NONE', ( #5732 ), #14095, .F. ) ;
#3984=DIRECTION ( 'NONE',  ( -0.000000000000000000, -0.000000000000000000, -1.000000000000000000 ) ) ;
#3996=CARTESIAN_POINT ( 'NONE',  ( 111.6227766016837961, 7.610970684806392799E-15, 6.000000000000000000 ) ) ;
#4013=CARTESIAN_POINT ( 'NONE',  ( 32.66827876307085887, -1.833751565556681173, 2.999999999999999112 ) ) ;
#4015=ORIENTED_EDGE ( 'NONE', *, *, #10395, .T. ) ;
#4021=PRODUCT_DEFINITION_FORMATION_WITH_SPECIFIED_SOURCE ( 'ANY', '', #10699, .NOT_KNOWN. ) ;
#4036=AXIS2_PLACEMENT_3D ( 'NONE', #1469, #7080, #10612 ) ;
#4037=ADVANCED_FACE ( 'NONE', ( #12929 ), #11629, .F. ) ;
#4041=EDGE_CURVE ( 'NONE', #5949, #4081, #550, .T. ) ;
#4061=AXIS2_PLACEMENT_3D ( 'NONE', #11789, #14262, #3724 ) ;
#4075=CIRCLE ( 'NONE', #6272, 3.000000000000002665 ) ;
#4081=VERTEX_POINT ( 'NONE', #6107 ) ;
#4083=CARTESIAN_POINT ( 'NONE',  ( 0.3363705501000964215, -6.891763197764913862, 6.000000000000000000 ) ) ;
#4087=ORIENTED_EDGE ( 'NONE', *, *, #2915, .T. ) ;
#4093=AXIS2_PLACEMENT_3D ( 'NONE', #12482, #6644, #10024 ) ;
#4103=EDGE_CURVE ( 'NONE', #9731, #8563, #14324, .T. ) ;
#4115=CARTESIAN_POINT ( 'NONE',  ( 0.000000000000000000, 0.000000000000000000, 5.500000000000000000 ) ) ;
#4120=VECTOR ( 'NONE', #2044, 1000.000000000000000 ) ;
#4179=DIRECTION ( 'NONE',  ( 1.000000000000000000, 0.000000000000000000, 0.000000000000000000 ) ) ;
#4180=EDGE_LOOP ( 'NONE', ( #7200, #2987, #11360, #3326, #10873, #2419, #4855, #7458, #3718, #3091 ) ) ;
#4181=DIRECTION ( 'NONE',  ( -0.5416238976136773520, 0.8406209333187990573, 0.000000000000000000 ) ) ;
#4182=FACE_OUTER_BOUND ( 'NONE', #13765, .T. ) ;
#4187=ORIENTED_EDGE ( 'NONE', *, *, #8071, .F. ) ;
#4193=ORIENTED_EDGE ( 'NONE', *, *, #9625, .F. ) ;
#4209=ORIENTED_EDGE ( 'NONE', *, *, #10286, .T. ) ;
#4223=EDGE_CURVE ( 'NONE', #13724, #5313, #11243, .T. ) ;
#4224=VERTEX_POINT ( 'NONE', #5424 ) ;
#4229=CYLINDRICAL_SURFACE ( 'NONE', #14667, 3.000000000000002665 ) ;
#4245=ORIENTED_EDGE ( 'NONE', *, *, #2287, .T. ) ;
#4247=ORIENTED_EDGE ( 'NONE', *, *, #9002, .T. ) ;
#4259=ORIENTED_EDGE ( 'NONE', *, *, #6450, .T. ) ;
#4270=ORIENTED_EDGE ( 'NONE', *, *, #1734, .F. ) ;
#4272=CARTESIAN_POINT ( 'NONE',  ( 101.6227766016837819, -9.999999999999994671, 6.000000000000000000 ) ) ;
#4309=DIRECTION ( 'NONE',  ( 0.000000000000000000, 0.000000000000000000, -1.000000000000000000 ) ) ;
#4325=EDGE_CURVE ( 'NONE', #1482, #14436, #9385, .T. ) ;
#4327=VECTOR ( 'NONE', #6445, 1000.000000000000000 ) ;
#4330=CARTESIAN_POINT ( 'NONE',  ( 15.21482963846748504, 16.90833299098317610, -131.1575142076926852 ) ) ;
#4333=CARTESIAN_POINT ( 'NONE',  ( 88.84370878116858705, 10.64188714589527507, 2.999999999999999112 ) ) ;
#4345=DIRECTION ( 'NONE',  ( -0.2314933715733012987, 0.9728364810787194505, 0.000000000000000000 ) ) ;
#4349=AXIS2_PLACEMENT_3D ( 'NONE', #12896, #11824, #289 ) ;
#4354=VERTEX_POINT ( 'NONE', #12768 ) ;
#4367=VECTOR ( 'NONE', #5882, 1000.000000000000000 ) ;
#4393=ORIENTED_EDGE ( 'NONE', *, *, #11078, .F. ) ;
#4398=ORIENTED_EDGE ( 'NONE', *, *, #1732, .T. ) ;
#4403=ORIENTED_EDGE ( 'NONE', *, *, #11078, .T. ) ;
#4417=AXIS2_PLACEMENT_3D ( 'NONE', #15063, #4309, #1929 ) ;
#4426=SURFACE_SIDE_STYLE ('',( #2029 ) ) ;
#4427=CARTESIAN_POINT ( 'NONE',  ( 80.00000000000000000, 0.000000000000000000, 6.000000000000000000 ) ) ;
#4430=CARTESIAN_POINT ( 'NONE',  ( 19.25177984293775069, 7.759396820770414926, 6.000000000000000000 ) ) ;
#4439=PLANE ( 'NONE',  #14685 ) ;
#4460=ORIENTED_EDGE ( 'NONE', *, *, #7701, .F. ) ;
#4462=LINE ( 'NONE', #5761, #5528 ) ;
#4463=CARTESIAN_POINT ( 'NONE',  ( 60.61028236725008611, -31.15713940066885712, 6.000000000000000000 ) ) ;
#4481=ORIENTED_EDGE ( 'NONE', *, *, #12890, .F. ) ;
#4482=DIRECTION ( 'NONE',  ( 1.000000000000000000, 0.000000000000000000, 0.000000000000000000 ) ) ;
#4484=CIRCLE ( 'NONE', #6438, 3.000000000000002665 ) ;
#4486=EDGE_CURVE ( 'NONE', #13724, #14414, #12366, .T. ) ;
#4487=ORIENTED_EDGE ( 'NONE', *, *, #14935, .T. ) ;
#4500=CYLINDRICAL_SURFACE ( 'NONE', #3536, 20.00000000000000000 ) ;
#4507=LINE ( 'NONE', #12569, #4120 ) ;
#4516=DIRECTION ( 'NONE',  ( -1.000000000000000000, 0.000000000000000000, -0.000000000000000000 ) ) ;
#4525=VECTOR ( 'NONE', #5265, 1000.000000000000000 ) ;
#4545=ADVANCED_FACE ( 'NONE', ( #45, #8357 ), #8067, .T. ) ;
#4548=VERTEX_POINT ( 'NONE', #11808 ) ;
#4555=CARTESIAN_POINT ( 'NONE',  ( 13.28797974610714761, -21.11867004231547540, -131.1575142076926852 ) ) ;
#4578=DIRECTION ( 'NONE',  ( 0.000000000000000000, 0.000000000000000000, 1.000000000000000000 ) ) ;
#4595=CIRCLE ( 'NONE', #4093, 11.66666666666667318 ) ;
#4604=EDGE_CURVE ( 'NONE', #11133, #13658, #13056, .T. ) ;
#4613=VERTEX_POINT ( 'NONE', #117 ) ;
#4620=DIRECTION ( 'NONE',  ( 2.081668171172168513E-16, -1.000000000000000000, 0.000000000000000000 ) ) ;
#4643=VECTOR ( 'NONE', #14575, 1000.000000000000114 ) ;
#4661=CARTESIAN_POINT ( 'NONE',  ( 0.04387302227425587953, -0.8988970056815600573, 6.000000000000000000 ) ) ;
#4671=VECTOR ( 'NONE', #6930, 1000.000000000000114 ) ;
#4678=VERTEX_POINT ( 'NONE', #4994 ) ;
#4688=ORIENTED_EDGE ( 'NONE', *, *, #12890, .T. ) ;
#4701=DIRECTION ( 'NONE',  ( 1.000000000000000000, 0.000000000000000000, 0.000000000000000000 ) ) ;
#4710=DIRECTION ( 'NONE',  ( -0.000000000000000000, -0.000000000000000000, -1.000000000000000000 ) ) ;
#4714=EDGE_CURVE ( 'NONE', #11238, #2991, #1361, .T. ) ;
#4716=CARTESIAN_POINT ( 'NONE',  ( 56.98919079003883326, 3.953582723775848962, 2.999999999999999112 ) ) ;
#4729=CARTESIAN_POINT ( 'NONE',  ( 84.00000000000000000, 0.000000000000000000, -131.1575142076926852 ) ) ;
#4740=CARTESIAN_POINT ( 'NONE',  ( 98.33955663538051795, 3.898681236723621879, 2.999999999999999112 ) ) ;
#4761=CARTESIAN_POINT ( 'NONE',  ( 101.4858053992934401, 0.9022481406819604643, 2.999999999999999112 ) ) ;
#4799=ORIENTED_EDGE ( 'NONE', *, *, #7701, .T. ) ;
#4805=CARTESIAN_POINT ( 'NONE',  ( 75.68384697807671557, 11.35494834827056110, 2.999999999999999112 ) ) ;
#4810=CARTESIAN_POINT ( 'NONE',  ( 14.40394475573011945, -10.79473832354794460, 22.47056274847713908 ) ) ;
#4827=ORIENTED_EDGE ( 'NONE', *, *, #2811, .F. ) ;
#4851=ADVANCED_FACE ( 'NONE', ( #6432 ), #8816, .F. ) ;
#4854=ORIENTED_EDGE ( 'NONE', *, *, #12731, .T. ) ;
#4855=ORIENTED_EDGE ( 'NONE', *, *, #8911, .T. ) ;
#4858=AXIS2_PLACEMENT_3D ( 'NONE', #4810, #2339, #10634 ) ;
#4866=AXIS2_PLACEMENT_3D ( 'NONE', #7380, #13514, #1523 ) ;
#4867=EDGE_CURVE ( 'NONE', #9019, #5489, #13232, .T. ) ;
#4868=EDGE_CURVE ( 'NONE', #5535, #7552, #15217, .T. ) ;
#4872=CARTESIAN_POINT ( 'NONE',  ( 86.17559721729969624, 12.01344854909570259, 2.999999999999999112 ) ) ;
#4875=ORIENTED_EDGE ( 'NONE', *, *, #11530, .F. ) ;
#4885=CARTESIAN_POINT ( 'NONE',  ( 3.321103546710217014, -13.95673088054953581, 6.000000000000000000 ) ) ;
#4887=AXIS2_PLACEMENT_3D ( 'NONE', #6570, #11172, #10462 ) ;
#4901=DIRECTION ( 'NONE',  ( -1.000000000000000000, 0.000000000000000000, 0.000000000000000000 ) ) ;
#4936=FACE_BOUND ( 'NONE', #2713, .T. ) ;
#4945=DIRECTION ( 'NONE',  ( 0.4571871344001384174, 0.8893705212896307888, -0.000000000000000000 ) ) ;
#4946=ORIENTED_EDGE ( 'NONE', *, *, #2915, .F. ) ;
#4959=DIRECTION ( 'NONE',  ( -0.000000000000000000, -0.000000000000000000, 1.000000000000000000 ) ) ;
#4960=CARTESIAN_POINT ( 'NONE',  ( 67.23404255319148604, 28.93147646537027384, 3.000000000000002665 ) ) ;
#4994=CARTESIAN_POINT ( 'NONE',  ( 8.403944755730119454, -10.79473832354794460, 3.000000000000000000 ) ) ;
#5000=ORIENTED_EDGE ( 'NONE', *, *, #11497, .F. ) ;
#5008=ORIENTED_EDGE ( 'NONE', *, *, #8213, .F. ) ;
#5009=VERTEX_POINT ( 'NONE', #3354 ) ;
#5014=CARTESIAN_POINT ( 'NONE',  ( 1.006169830977205581, -4.228366069762346413, 6.000000000000000000 ) ) ;
#5021=ORIENTED_EDGE ( 'NONE', *, *, #2329, .F. ) ;
#5027=AXIS2_PLACEMENT_3D ( 'NONE', #1411, #12240, #5035 ) ;
#5030=CARTESIAN_POINT ( 'NONE',  ( 80.00000000000000000, 0.000000000000000000, -131.1575142076926852 ) ) ;
#5035=DIRECTION ( 'NONE',  ( 1.000000000000000000, 0.000000000000000000, 0.000000000000000000 ) ) ;
#5038=EDGE_LOOP ( 'NONE', ( #7408, #6919 ) ) ;
#5053=CARTESIAN_POINT ( 'NONE',  ( 80.82762530298222714, -9.999999999999994671, 3.000000000000002665 ) ) ;
#5058=AXIS2_PLACEMENT_3D ( 'NONE', #2485, #3702, #158 ) ;
#5072=VECTOR ( 'NONE', #12355, 1000.000000000000000 ) ;
#5087=ORIENTED_EDGE ( 'NONE', *, *, #7030, .F. ) ;
#5094=CARTESIAN_POINT ( 'NONE',  ( 14.40394475573011945, -10.79473832354794460, 6.000000000000000000 ) ) ;
#5112=AXIS2_PLACEMENT_3D ( 'NONE', #9450, #1382, #2470 ) ;
#5114=DIRECTION ( 'NONE',  ( 1.000000000000000000, 0.000000000000000000, 0.000000000000000000 ) ) ;
#5129=EDGE_LOOP ( 'NONE', ( #4270, #9964, #15197, #4403 ) ) ;
#5147=CIRCLE ( 'NONE', #6607, 2.999999999999988898 ) ;
#5163=CARTESIAN_POINT ( 'NONE',  ( 55.83172393217232354, 8.817765129169439220, 2.999999999999999112 ) ) ;
#5168=ORIENTED_EDGE ( 'NONE', *, *, #12465, .F. ) ;
#5169=ORIENTED_EDGE ( 'NONE', *, *, #5705, .F. ) ;
#5178=EDGE_CURVE ( 'NONE', #9228, #2441, #10871, .T. ) ;
#5182=CIRCLE ( 'NONE', #7087, 6.000000000000000000 ) ;
#5191=DIRECTION ( 'NONE',  ( 1.000000000000000000, 0.000000000000000000, 0.000000000000000000 ) ) ;
#5198=DIRECTION ( 'NONE',  ( 0.000000000000000000, 0.000000000000000000, 1.000000000000000000 ) ) ;
#5201=DIRECTION ( 'NONE',  ( -0.000000000000000000, -0.000000000000000000, 1.000000000000000000 ) ) ;
#5212=LINE ( 'NONE', #6347, #14289 ) ;
#5214=ORIENTED_EDGE ( 'NONE', *, *, #4103, .T. ) ;
#5216=VERTEX_POINT ( 'NONE', #5709 ) ;
#5224=DIRECTION ( 'NONE',  ( -0.000000000000000000, -0.000000000000000000, -1.000000000000000000 ) ) ;
#5226=ORIENTED_EDGE ( 'NONE', *, *, #8918, .T. ) ;
#5243=CARTESIAN_POINT ( 'NONE',  ( 91.12964445316929130, 15.08873975234342701, 6.000000000000000000 ) ) ;
#5255=EDGE_LOOP ( 'NONE', ( #12377, #5345, #6749, #2187 ) ) ;
#5265=DIRECTION ( 'NONE',  ( -0.000000000000000000, -0.000000000000000000, -1.000000000000000000 ) ) ;
#5266=CARTESIAN_POINT ( 'NONE',  ( 72.49759028996471955, 17.18292470770558822, 2.999999999999999112 ) ) ;
#5270=EDGE_LOOP ( 'NONE', ( #12158, #9617, #11837, #8392 ) ) ;
#5272=CARTESIAN_POINT ( 'NONE',  ( -4.000000000000000000, 0.000000000000000000, 6.000000000000000000 ) ) ;
#5277=CARTESIAN_POINT ( 'NONE',  ( 76.00000000000000000, 4.898587196589420717E-16, -131.1575142076926852 ) ) ;
#5284=VERTEX_POINT ( 'NONE', #3098 ) ;
#5304=ORIENTED_EDGE ( 'NONE', *, *, #8552, .F. ) ;
#5305=CARTESIAN_POINT ( 'NONE',  ( 0.000000000000000000, 0.000000000000000000, 6.000000000000000000 ) ) ;
#5309=VERTEX_POINT ( 'NONE', #10085 ) ;
#5313=VERTEX_POINT ( 'NONE', #15012 ) ;
#5325=CARTESIAN_POINT ( 'NONE',  ( 14.40394475573011945, -10.79473832354794460, 5.500000000000000000 ) ) ;
#5331=EDGE_CURVE ( 'NONE', #13989, #4548, #3401, .T. ) ;
#5332=EDGE_LOOP ( 'NONE', ( #7589, #14128 ) ) ;
#5336=CARTESIAN_POINT ( 'NONE',  ( -9.999999999999998224, 0.000000000000000000, 3.000000000000002665 ) ) ;
#5339=UNCERTAINTY_MEASURE_WITH_UNIT (LENGTH_MEASURE( 1.000000000000000082E-05 ), #10257, 'distance_accuracy_value', 'NONE');
#5343=DIRECTION ( 'NONE',  ( -0.000000000000000000, -0.000000000000000000, 1.000000000000000000 ) ) ;
#5345=ORIENTED_EDGE ( 'NONE', *, *, #10742, .F. ) ;
#5363=CARTESIAN_POINT ( 'NONE',  ( 13.28797974610715116, -21.11867004231547540, 6.000000000000000000 ) ) ;
#5367=( GEOMETRIC_REPRESENTATION_CONTEXT ( 3 ) GLOBAL_UNCERTAINTY_ASSIGNED_CONTEXT ( ( #11007 ) ) GLOBAL_UNIT_ASSIGNED_CONTEXT ( ( #253, #12255, #1655 ) ) REPRESENTATION_CONTEXT ( 'NONE', 'WORKASPACE' ) );
#5371=CIRCLE ( 'NONE', #9036, 4.999999999999997335 ) ;
#5388=LINE ( 'NONE', #2986, #14353 ) ;
#5393=CARTESIAN_POINT ( 'NONE',  ( 56.98919079003883326, 3.953582723775848962, 2.999999999999999112 ) ) ;
#5399=CARTESIAN_POINT ( 'NONE',  ( 80.82762530298222714, -9.999999999999994671, 6.000000000000000000 ) ) ;
#5424=CARTESIAN_POINT ( 'NONE',  ( 93.34550147531103903, 3.654933296868752457, 2.999999999999999112 ) ) ;
#5429=VERTEX_POINT ( 'NONE', #14001 ) ;
#5470=EDGE_CURVE ( 'NONE', #3838, #214, #12506, .T. ) ;
#5475=CARTESIAN_POINT ( 'NONE',  ( 79.18363542992867110, -10.13606076167855008, 6.000000000000000000 ) ) ;
#5489=VERTEX_POINT ( 'NONE', #7317 ) ;
#5508=VERTEX_POINT ( 'NONE', #8535 ) ;
#5515=ORIENTED_EDGE ( 'NONE', *, *, #5470, .T. ) ;
#5517=AXIS2_PLACEMENT_3D ( 'NONE', #13136, #1470, #8753 ) ;
#5518=CARTESIAN_POINT ( 'NONE',  ( -9.999999999999998224, -1.390791565672605534, 3.000000000000002665 ) ) ;
#5528=VECTOR ( 'NONE', #13981, 1000.000000000000000 ) ;
#5534=CARTESIAN_POINT ( 'NONE',  ( -9.999999999999998224, 0.000000000000000000, 3.000000000000002665 ) ) ;
#5535=VERTEX_POINT ( 'NONE', #5243 ) ;
#5564=ORIENTED_EDGE ( 'NONE', *, *, #15030, .T. ) ;
#5566=CARTESIAN_POINT ( 'NONE',  ( 83.50748565343083385, 13.38500995229612478, 2.999999999999999112 ) ) ;
#5571=DIRECTION ( 'NONE',  ( 1.000000000000000000, 0.000000000000000000, 0.000000000000000000 ) ) ;
#5576=AXIS2_PLACEMENT_3D ( 'NONE', #3268, #5590, #9116 ) ;
#5577=( NAMED_UNIT ( * ) SI_UNIT ( $, .STERADIAN. ) SOLID_ANGLE_UNIT ( ) );
#5590=DIRECTION ( 'NONE',  ( -0.8406209333187997235, -0.5416238976136762417, 0.000000000000000000 ) ) ;
#5591=ORIENTED_EDGE ( 'NONE', *, *, #14084, .T. ) ;
#5597=CARTESIAN_POINT ( 'NONE',  ( 55.83172393217232354, 8.817765129169439220, 6.000000000000000000 ) ) ;
#5606=CARTESIAN_POINT ( 'NONE',  ( 8.403944755730119454, -10.79473832354794460, 5.500000000000001776 ) ) ;
#5620=DIRECTION ( 'NONE',  ( -0.4571871344001416926, -0.8893705212896291235, 0.000000000000000000 ) ) ;
#5625=EDGE_CURVE ( 'NONE', #5216, #2895, #3426, .T. ) ;
#5640=CIRCLE ( 'NONE', #11259, 9.999999999999994671 ) ;
#5656=DIRECTION ( 'NONE',  ( 0.000000000000000000, 0.000000000000000000, 1.000000000000000000 ) ) ;
#5662=CARTESIAN_POINT ( 'NONE',  ( 98.48580539929344013, 0.9022481406819604643, 2.999999999999999112 ) ) ;
#5685=ORIENTED_EDGE ( 'NONE', *, *, #4325, .T. ) ;
#5705=EDGE_CURVE ( 'NONE', #4548, #5009, #13743, .T. ) ;
#5709=CARTESIAN_POINT ( 'NONE',  ( 86.00000000000000000, 7.347880794884117764E-16, 3.000000000000000000 ) ) ;
#5732=FACE_OUTER_BOUND ( 'NONE', #11462, .T. ) ;
#5748=DIRECTION ( 'NONE',  ( 1.000000000000000000, 0.000000000000000000, 0.000000000000000000 ) ) ;
#5754=VECTOR ( 'NONE', #3168, 1000.000000000000000 ) ;
#5761=CARTESIAN_POINT ( 'NONE',  ( 98.63205416320636232, -2.094184955359725375, 2.999999999999999112 ) ) ;
#5765=CARTESIAN_POINT ( 'NONE',  ( 33.82574562093736859, -6.697933970950280091, 2.999999999999999112 ) ) ;
#5776=ORIENTED_EDGE ( 'NONE', *, *, #5813, .F. ) ;
#5777=ORIENTED_EDGE ( 'NONE', *, *, #13886, .F. ) ;
#5781=DIRECTION ( 'NONE',  ( 0.000000000000000000, 0.000000000000000000, 1.000000000000000000 ) ) ;
#5782=PLANE ( 'NONE',  #11714 ) ;
#5788=CARTESIAN_POINT ( 'NONE',  ( 80.82762530298222714, -19.99999999999999645, 6.000000000000005329 ) ) ;
#5790=EDGE_CURVE ( 'NONE', #10601, #7097, #12745, .T. ) ;
#5793=CARTESIAN_POINT ( 'NONE',  ( -10.00000000000000000, -2.081668171172168513E-15, 6.000000000000000000 ) ) ;
#5813=EDGE_CURVE ( 'NONE', #15059, #6090, #9433, .T. ) ;
#5818=EDGE_CURVE ( 'NONE', #13731, #555, #11810, .T. ) ;
#5819=VECTOR ( 'NONE', #3896, 1000.000000000000114 ) ;
#5840=DIRECTION ( 'NONE',  ( 1.000000000000000000, 0.000000000000000000, 0.000000000000000000 ) ) ;
#5847=EDGE_CURVE ( 'NONE', #7404, #5216, #2908, .T. ) ;
#5848=ORIENTED_EDGE ( 'NONE', *, *, #14084, .F. ) ;
#5863=CARTESIAN_POINT ( 'NONE',  ( 67.45386469005195806, 13.93318132202354676, 6.000000000000000000 ) ) ;
#5874=DIRECTION ( 'NONE',  ( 0.000000000000000000, 0.000000000000000000, 1.000000000000000000 ) ) ;
#5882=DIRECTION ( 'NONE',  ( -0.000000000000000000, -0.000000000000000000, -1.000000000000000000 ) ) ;
#5890=ORIENTED_EDGE ( 'NONE', *, *, #9480, .T. ) ;
#5900=FACE_OUTER_BOUND ( 'NONE', #13110, .T. ) ;
#5927=ORIENTED_EDGE ( 'NONE', *, *, #9364, .T. ) ;
#5929=DIRECTION ( 'NONE',  ( -1.000000000000000000, 0.000000000000000000, -0.000000000000000000 ) ) ;
#5932=DIRECTION ( 'NONE',  ( 1.000000000000000000, 0.000000000000000000, 0.000000000000000000 ) ) ;
#5944=AXIS2_PLACEMENT_3D ( 'NONE', #9284, #11646, #3435 ) ;
#5949=VERTEX_POINT ( 'NONE', #2600 ) ;
#5966=DIRECTION ( 'NONE',  ( -1.000000000000000000, 0.000000000000000000, 0.000000000000000000 ) ) ;
#5980=EDGE_LOOP ( 'NONE', ( #5214, #14704, #1098, #6527, #1808 ) ) ;
#5985=FACE_OUTER_BOUND ( 'NONE', #8560, .T. ) ;
#5987=ORIENTED_EDGE ( 'NONE', *, *, #5331, .F. ) ;
#6005=LINE ( 'NONE', #7160, #14903 ) ;
#6009=VECTOR ( 'NONE', #5201, 1000.000000000000000 ) ;
#6015=EDGE_CURVE ( 'NONE', #9599, #9731, #12695, .T. ) ;
#6047=EDGE_LOOP ( 'NONE', ( #9676, #10865, #2341, #1976 ) ) ;
#6054=CARTESIAN_POINT ( 'NONE',  ( 0.000000000000000000, 0.000000000000000000, 5.500000000000000000 ) ) ;
#6071=VECTOR ( 'NONE', #372, 1000.000000000000000 ) ;
#6078=DIRECTION ( 'NONE',  ( -1.000000000000000000, 0.000000000000000000, 0.000000000000000000 ) ) ;
#6086=VECTOR ( 'NONE', #10089, 1000.000000000000000 ) ;
#6090=VERTEX_POINT ( 'NONE', #9411 ) ;
#6096=VECTOR ( 'NONE', #326, 1000.000000000000000 ) ;
#6107=CARTESIAN_POINT ( 'NONE',  ( 72.49759028996471955, 17.18292470770558822, 6.000000000000000000 ) ) ;
#6109=DIRECTION ( 'NONE',  ( 0.9988110320138940956, 0.04874958797097354857, 0.000000000000000000 ) ) ;
#6120=DIRECTION ( 'NONE',  ( -0.04874958797097372204, 0.9988110320138942066, 0.000000000000000000 ) ) ;
#6150=CARTESIAN_POINT ( 'NONE',  ( 4.000000000000000000, 4.898587196589412829E-16, 6.000000000000000000 ) ) ;
#6158=EDGE_CURVE ( 'NONE', #8579, #13244, #13756, .T. ) ;
#6159=EDGE_CURVE ( 'NONE', #14461, #6202, #9281, .T. ) ;
#6161=ORIENTED_EDGE ( 'NONE', *, *, #8722, .F. ) ;
#6180=LINE ( 'NONE', #2793, #14854 ) ;
#6182=ORIENTED_EDGE ( 'NONE', *, *, #2784, .T. ) ;
#6187=DIRECTION ( 'NONE',  ( 0.000000000000000000, 0.000000000000000000, 1.000000000000000000 ) ) ;
#6197=LINE ( 'NONE', #14578, #5819 ) ;
#6198=EDGE_CURVE ( 'NONE', #1136, #2216, #5182, .T. ) ;
#6200=AXIS2_PLACEMENT_3D ( 'NONE', #2109, #13566, #7810 ) ;
#6202=VERTEX_POINT ( 'NONE', #5053 ) ;
#6210=AXIS2_PLACEMENT_3D ( 'NONE', #3562, #8249, #1560 ) ;
#6221=ORIENTED_EDGE ( 'NONE', *, *, #9541, .T. ) ;
#6224=LINE ( 'NONE', #14763, #6071 ) ;
#6230=DIRECTION ( 'NONE',  ( 0.9988110320138940956, 0.04874958797097353469, -0.000000000000000000 ) ) ;
#6250=AXIS2_PLACEMENT_3D ( 'NONE', #8516, #1526, #1830 ) ;
#6262=VECTOR ( 'NONE', #7778, 1000.000000000000000 ) ;
#6265=CARTESIAN_POINT ( 'NONE',  ( 93.34550147531103903, 3.654933296868752457, 2.999999999999999112 ) ) ;
#6267=DIRECTION ( 'NONE',  ( -0.4036950204470272086, 0.9148936170212765839, 0.000000000000000000 ) ) ;
#6272=AXIS2_PLACEMENT_3D ( 'NONE', #12549, #8013, #5571 ) ;
#6276=ADVANCED_FACE ( 'NONE', ( #7426 ), #186, .F. ) ;
#6279=CARTESIAN_POINT ( 'NONE',  ( 55.83172393217232354, 8.817765129169439220, 2.999999999999999112 ) ) ;
#6288=ORIENTED_EDGE ( 'NONE', *, *, #1570, .T. ) ;
#6289=DIRECTION ( 'NONE',  ( 1.000000000000000000, 0.000000000000000000, 0.000000000000000000 ) ) ;
#6293=EDGE_CURVE ( 'NONE', #2630, #9228, #5640, .T. ) ;
#6296=EDGE_CURVE ( 'NONE', #4224, #8100, #10872, .T. ) ;
#6308=AXIS2_PLACEMENT_3D ( 'NONE', #4716, #9692, #9383 ) ;
#6313=VECTOR ( 'NONE', #15042, 1000.000000000000000 ) ;
#6323=CIRCLE ( 'NONE', #3620, 4.999999999999997335 ) ;
#6328=CARTESIAN_POINT ( 'NONE',  ( 33.82574562093736148, -6.697933970950280091, 6.000000000000000000 ) ) ;
#6344=VECTOR ( 'NONE', #2281, 1000.000000000000000 ) ;
#6345=ORIENTED_EDGE ( 'NONE', *, *, #5178, .F. ) ;
#6346=CARTESIAN_POINT ( 'NONE',  ( -9.999999999999992895, -25.00000000000000000, 3.000000000000002665 ) ) ;
#6347=CARTESIAN_POINT ( 'NONE',  ( 93.63799900313688340, -2.337932895214617890, 2.999999999999999112 ) ) ;
#6354=CIRCLE ( 'NONE', #6606, 2.999999999999975131 ) ;
#6374=CARTESIAN_POINT ( 'NONE',  ( 79.18363542992865689, -10.13606076167855541, 6.000000000000005329 ) ) ;
#6387=VERTEX_POINT ( 'NONE', #4430 ) ;
#6408=DIRECTION ( 'NONE',  ( -0.000000000000000000, -0.000000000000000000, 1.000000000000000000 ) ) ;
#6409=LINE ( 'NONE', #8859, #6009 ) ;
#6410=VERTEX_POINT ( 'NONE', #10032 ) ;
#6415=DIRECTION ( 'NONE',  ( 0.000000000000000000, 0.000000000000000000, 1.000000000000000000 ) ) ;
#6432=FACE_OUTER_BOUND ( 'NONE', #7421, .T. ) ;
#6433=ADVANCED_FACE ( 'NONE', ( #8797 ), #7882, .F. ) ;
#6438=AXIS2_PLACEMENT_3D ( 'NONE', #5662, #10184, #3265 ) ;
#6445=DIRECTION ( 'NONE',  ( -0.000000000000000000, -0.000000000000000000, 1.000000000000000000 ) ) ;
#6450=EDGE_CURVE ( 'NONE', #3757, #14414, #5147, .T. ) ;
#6452=EDGE_CURVE ( 'NONE', #6485, #15027, #6323, .T. ) ;
#6476=DIRECTION ( 'NONE',  ( 0.4571871344001383619, 0.8893705212896307888, 0.000000000000000000 ) ) ;
#6485=VERTEX_POINT ( 'NONE', #10400 ) ;
#6488=DIRECTION ( 'NONE',  ( 1.000000000000000000, 0.000000000000000000, -0.000000000000000000 ) ) ;
#6506=CARTESIAN_POINT ( 'NONE',  ( 32.66827876307085887, -1.833751565556681173, 6.000000000000000000 ) ) ;
#6507=EDGE_CURVE ( 'NONE', #5489, #6410, #1253, .T. ) ;
#6516=FACE_OUTER_BOUND ( 'NONE', #14994, .T. ) ;
#6523=ADVANCED_FACE ( 'NONE', ( #3263 ), #6797, .F. ) ;
#6524=FACE_OUTER_BOUND ( 'NONE', #13859, .T. ) ;
#6527=ORIENTED_EDGE ( 'NONE', *, *, #1527, .T. ) ;
#6551=AXIS2_PLACEMENT_3D ( 'NONE', #518, #14462, #7538 ) ;
#6570=CARTESIAN_POINT ( 'NONE',  ( 0.000000000000000000, 0.000000000000000000, 3.000000000000000000 ) ) ;
#6577=COLOUR_RGB ( '',0.8941176470588234615, 0.8941176470588234615, 0.8941176470588234615 ) ;
#6582=VECTOR ( 'NONE', #14204, 1000.000000000000114 ) ;
#6590=AXIS2_PLACEMENT_3D ( 'NONE', #2001, #1925, #6758 ) ;
#6592=DIRECTION ( 'NONE',  ( 0.8406209333187990573, 0.5416238976136773520, 0.000000000000000000 ) ) ;
#6596=AXIS2_PLACEMENT_3D ( 'NONE', #491, #6267, #8643 ) ;
#6598=DIRECTION ( 'NONE',  ( 0.000000000000000000, 0.000000000000000000, -1.000000000000000000 ) ) ;
#6602=DIRECTION ( 'NONE',  ( 0.000000000000000000, 0.000000000000000000, -1.000000000000000000 ) ) ;
#6606=AXIS2_PLACEMENT_3D ( 'NONE', #10513, #14036, #14113 ) ;
#6607=AXIS2_PLACEMENT_3D ( 'NONE', #12558, #7578, #2033 ) ;
#6610=ORIENTED_EDGE ( 'NONE', *, *, #11532, .F. ) ;
#6619=DIRECTION ( 'NONE',  ( 0.000000000000000000, 0.000000000000000000, 1.000000000000000000 ) ) ;
#6622=ADVANCED_FACE ( 'NONE', ( #12844 ), #7019, .F. ) ;
#6638=AXIS2_PLACEMENT_3D ( 'NONE', #11517, #6619, #994 ) ;
#6644=DIRECTION ( 'NONE',  ( -0.000000000000000000, -0.000000000000000000, -1.000000000000000000 ) ) ;
#6650=ADVANCED_FACE ( 'NONE', ( #2720 ), #12001, .F. ) ;
#6658=LINE ( 'NONE', #2112, #2151 ) ;
#6690=ORIENTED_EDGE ( 'NONE', *, *, #13311, .T. ) ;
#6694=ORIENTED_EDGE ( 'NONE', *, *, #8303, .F. ) ;
#6714=PRESENTATION_STYLE_ASSIGNMENT (( #13718 ) ) ;
#6717=ORIENTED_EDGE ( 'NONE', *, *, #10701, .T. ) ;
#6718=CARTESIAN_POINT ( 'NONE',  ( 56.98919079003883326, 3.953582723775848962, 6.000000000000000000 ) ) ;
#6726=PLANE ( 'NONE',  #5576 ) ;
#6749=ORIENTED_EDGE ( 'NONE', *, *, #340, .F. ) ;
#6752=ORIENTED_EDGE ( 'NONE', *, *, #8413, .F. ) ;
#6758=DIRECTION ( 'NONE',  ( 1.000000000000000000, 0.000000000000000000, 0.000000000000000000 ) ) ;
#6759=CARTESIAN_POINT ( 'NONE',  ( -9.999999999999998224, 0.000000000000000000, 6.000000000000000000 ) ) ;
#6768=CARTESIAN_POINT ( 'NONE',  ( 67.23404255319148604, 28.93147646537027384, 6.000000000000000000 ) ) ;
#6777=EDGE_CURVE ( 'NONE', #8563, #108, #714, .T. ) ;
#6778=DIRECTION ( 'NONE',  ( 0.9863939238321436376, 0.1643989873053573192, 0.000000000000000000 ) ) ;
#6789=ORIENTED_EDGE ( 'NONE', *, *, #4867, .T. ) ;
#6795=EDGE_LOOP ( 'NONE', ( #8648, #1706, #12639, #470 ) ) ;
#6797=CYLINDRICAL_SURFACE ( 'NONE', #926, 9.999999999999994671 ) ;
#6806=ORIENTED_EDGE ( 'NONE', *, *, #2811, .T. ) ;
#6830=ORIENTED_EDGE ( 'NONE', *, *, #8239, .F. ) ;
#6854=ADVANCED_FACE ( 'NONE', ( #4182 ), #8853, .F. ) ;
#6872=DIRECTION ( 'NONE',  ( 0.000000000000000000, 0.000000000000000000, 1.000000000000000000 ) ) ;
#6886=CARTESIAN_POINT ( 'NONE',  ( 75.20570977803312473, 12.97982004111159959, 2.999999999999999112 ) ) ;
#6894=CARTESIAN_POINT ( 'NONE',  ( 86.00000000000000000, 7.347880794884117764E-16, 5.500000000000000000 ) ) ;
#6906=EDGE_CURVE ( 'NONE', #6954, #5429, #12612, .T. ) ;
#6913=CARTESIAN_POINT ( 'NONE',  ( 75.20570977803312473, 12.97982004111159959, 2.999999999999999112 ) ) ;
#6914=PLANE ( 'NONE',  #6978 ) ;
#6915=VECTOR ( 'NONE', #6476, 1000.000000000000114 ) ;
#6919=ORIENTED_EDGE ( 'NONE', *, *, #5625, .F. ) ;
#6922=ORIENTED_EDGE ( 'NONE', *, *, #10233, .F. ) ;
#6930=DIRECTION ( 'NONE',  ( 0.5416238976136762417, -0.8406209333187997235, -0.000000000000000000 ) ) ;
#6933=ADVANCED_FACE ( 'NONE', ( #10670 ), #10386, .T. ) ;
#6944=VECTOR ( 'NONE', #10792, 1000.000000000000114 ) ;
#6954=VERTEX_POINT ( 'NONE', #10752 ) ;
#6978=AXIS2_PLACEMENT_3D ( 'NONE', #5765, #1225, #7064 ) ;
#6981=DIRECTION ( 'NONE',  ( -1.000000000000000000, 0.000000000000000000, 0.000000000000000000 ) ) ;
#6987=CYLINDRICAL_SURFACE ( 'NONE', #10222, 2.999999999999988898 ) ;
#7003=EDGE_LOOP ( 'NONE', ( #4799, #7906, #6830, #10302 ) ) ;
#7016=EDGE_CURVE ( 'NONE', #4354, #4613, #937, .T. ) ;
#7019=PLANE ( 'NONE',  #2932 ) ;
#7023=ORIENTED_EDGE ( 'NONE', *, *, #14307, .T. ) ;
#7026=DIRECTION ( 'NONE',  ( 0.000000000000000000, 0.000000000000000000, 1.000000000000000000 ) ) ;
#7030=EDGE_CURVE ( 'NONE', #12603, #2895, #8819, .T. ) ;
#7033=EDGE_CURVE ( 'NONE', #4224, #7818, #13453, .T. ) ;
#7034=AXIS2_PLACEMENT_3D ( 'NONE', #11502, #7904, #5748 ) ;
#7037=DIRECTION ( 'NONE',  ( 1.000000000000000000, 0.000000000000000000, 0.000000000000000000 ) ) ;
#7041=AXIS2_PLACEMENT_3D ( 'NONE', #135, #12825, #5929 ) ;
#7045=DIRECTION ( 'NONE',  ( -0.000000000000000000, -0.000000000000000000, -1.000000000000000000 ) ) ;
#7051=ORIENTED_EDGE ( 'NONE', *, *, #2784, .F. ) ;
#7057=CARTESIAN_POINT ( 'NONE',  ( 75.68384697807671557, 11.35494834827056110, 6.000000000000000000 ) ) ;
#7064=DIRECTION ( 'NONE',  ( 0.9728364810787194505, 0.2314933715733012709, 0.000000000000000000 ) ) ;
#7069=AXIS2_PLACEMENT_3D ( 'NONE', #6054, #1218, #9427 ) ;
#7079=DIRECTION ( 'NONE',  ( -0.000000000000000000, -0.000000000000000000, -1.000000000000000000 ) ) ;
#7080=DIRECTION ( 'NONE',  ( 0.000000000000000000, -1.000000000000000000, 0.000000000000000000 ) ) ;
#7084=EDGE_LOOP ( 'NONE', ( #10105, #6345, #9863, #4393 ) ) ;
#7085=LINE ( 'NONE', #4083, #9006 ) ;
#7087=AXIS2_PLACEMENT_3D ( 'NONE', #8715, #13408, #2662 ) ;
#7097=VERTEX_POINT ( 'NONE', #7669 ) ;
#7109=ADVANCED_FACE ( 'NONE', ( #2982 ), #10823, .F. ) ;
#7116=CYLINDRICAL_SURFACE ( 'NONE', #4061, 3.000000000000002665 ) ;
#7146=CARTESIAN_POINT ( 'NONE',  ( 70.16198417812034904, 9.730076655429538590, 6.000000000000000000 ) ) ;
#7160=CARTESIAN_POINT ( 'NONE',  ( 65.94650549498813064, -33.90026220706954518, 6.000000000000000000 ) ) ;
#7165=ADVANCED_FACE ( 'NONE', ( #8737 ), #13433, .F. ) ;
#7188=FACE_OUTER_BOUND ( 'NONE', #12481, .T. ) ;
#7193=LINE ( 'NONE', #1346, #6344 ) ;
#7199=ADVANCED_FACE ( 'NONE', ( #13810, #6516 ), #8969, .T. ) ;
#7200=ORIENTED_EDGE ( 'NONE', *, *, #7892, .T. ) ;
#7207=EDGE_LOOP ( 'NONE', ( #3092, #13599, #596, #2578, #7023, #12724, #6717, #1682, #3617, #10173 ) ) ;
#7219=CIRCLE ( 'NONE', #10168, 6.000000000000000000 ) ;
#7229=CIRCLE ( 'NONE', #854, 5.999999999999999112 ) ;
#7239=VECTOR ( 'NONE', #3763, 1000.000000000000227 ) ;
#7250=AXIS2_PLACEMENT_3D ( 'NONE', #13697, #5781, #10460 ) ;
#7252=CARTESIAN_POINT ( 'NONE',  ( 0.000000000000000000, 0.000000000000000000, 6.000000000000000000 ) ) ;
#7264=DIRECTION ( 'NONE',  ( -1.000000000000000000, 0.000000000000000000, 0.000000000000000000 ) ) ;
#7269=PRODUCT_DEFINITION_SHAPE ( 'NONE', 'NONE',  #12917 ) ;
#7279=AXIS2_PLACEMENT_3D ( 'NONE', #12299, #2849, #12368 ) ;
#7300=CIRCLE ( 'NONE', #9739, 2.999999999999988898 ) ;
#7305=ORIENTED_EDGE ( 'NONE', *, *, #4714, .F. ) ;
#7312=CARTESIAN_POINT ( 'NONE',  ( 15.21482963846748504, 16.90833299098317610, 6.000000000000005329 ) ) ;
#7317=CARTESIAN_POINT ( 'NONE',  ( 5.999999999999999112, 7.347880794884118750E-16, 5.500000000000000000 ) ) ;
#7320=DIRECTION ( 'NONE',  ( -0.000000000000000000, -0.000000000000000000, 1.000000000000000000 ) ) ;
#7325=ORIENTED_EDGE ( 'NONE', *, *, #4041, .T. ) ;
#7335=ADVANCED_FACE ( 'NONE', ( #5900 ), #8189, .F. ) ;
#7342=ORIENTED_EDGE ( 'NONE', *, *, #11881, .F. ) ;
#7353=CARTESIAN_POINT ( 'NONE',  ( 0.000000000000000000, 0.000000000000000000, 0.000000000000000000 ) ) ;
#7380=CARTESIAN_POINT ( 'NONE',  ( 93.49175023922396122, 0.6585002008270834928, 2.999999999999999112 ) ) ;
#7396=LINE ( 'NONE', #5014, #14092 ) ;
#7404=VERTEX_POINT ( 'NONE', #6894 ) ;
#7407=EDGE_CURVE ( 'NONE', #7557, #13658, #7193, .T. ) ;
#7408=ORIENTED_EDGE ( 'NONE', *, *, #11141, .F. ) ;
#7409=DIRECTION ( 'NONE',  ( -0.000000000000000000, -0.000000000000000000, 1.000000000000000000 ) ) ;
#7413=LINE ( 'NONE', #4885, #8196 ) ;
#7414=EDGE_LOOP ( 'NONE', ( #2641, #7816, #9962, #14352, #13554 ) ) ;
#7421=EDGE_LOOP ( 'NONE', ( #3258, #6752, #10064, #247 ) ) ;
#7422=FACE_OUTER_BOUND ( 'NONE', #10294, .T. ) ;
#7426=FACE_OUTER_BOUND ( 'NONE', #7003, .T. ) ;
#7428=ADVANCED_FACE ( 'NONE', ( #3967 ), #13090, .T. ) ;
#7437=EDGE_CURVE ( 'NONE', #3359, #12316, #412, .T. ) ;
#7458=ORIENTED_EDGE ( 'NONE', *, *, #12652, .T. ) ;
#7475=ORIENTED_EDGE ( 'NONE', *, *, #2287, .F. ) ;
#7483=CIRCLE ( 'NONE', #855, 9.999999999999994671 ) ;
#7494=EDGE_LOOP ( 'NONE', ( #1913, #11792 ) ) ;
#7501=CIRCLE ( 'NONE', #12638, 4.000000000000000000 ) ;
#7523=CARTESIAN_POINT ( 'NONE',  ( 67.23404255319145761, 28.93147646537026318, -131.1575142076926852 ) ) ;
#7526=ORIENTED_EDGE ( 'NONE', *, *, #1393, .F. ) ;
#7529=DIRECTION ( 'NONE',  ( -0.000000000000000000, -0.000000000000000000, 1.000000000000000000 ) ) ;
#7538=DIRECTION ( 'NONE',  ( 1.000000000000000000, 0.000000000000000000, 0.000000000000000000 ) ) ;
#7551=STYLED_ITEM('',(#15258),#3822);
#7552=VERTEX_POINT ( 'NONE', #13259 ) ;
#7557=VERTEX_POINT ( 'NONE', #8490 ) ;
#7569=CYLINDRICAL_SURFACE ( 'NONE', #11204, 4.999999999999997335 ) ;
#7577=FACE_BOUND ( 'NONE', #1551, .T. ) ;
#7578=DIRECTION ( 'NONE',  ( 0.000000000000000000, 0.000000000000000000, 1.000000000000000000 ) ) ;
#7589=ORIENTED_EDGE ( 'NONE', *, *, #511, .T. ) ;
#7591=AXIS2_PLACEMENT_3D ( 'NONE', #7252, #314, #2555 ) ;
#7601=ORIENTED_EDGE ( 'NONE', *, *, #3878, .T. ) ;
#7612=ORIENTED_EDGE ( 'NONE', *, *, #7437, .F. ) ;
#7626=EDGE_LOOP ( 'NONE', ( #11631, #3180, #11821, #7342 ) ) ;
#7628=LINE ( 'NONE', #5336, #6262 ) ;
#7630=PRODUCT_DEFINITION_CONTEXT ( 'detailed design', #13013, 'design' ) ;
#7648=FACE_OUTER_BOUND ( 'NONE', #7207, .T. ) ;
#7669=CARTESIAN_POINT ( 'NONE',  ( 75.20570977803312473, 12.97982004111160315, 6.000000000000000000 ) ) ;
#7685=ADVANCED_FACE ( 'NONE', ( #11399 ), #12330, .T. ) ;
#7696=ORIENTED_EDGE ( 'NONE', *, *, #6198, .T. ) ;
#7701=EDGE_CURVE ( 'NONE', #2991, #8100, #15031, .T. ) ;
#7708=DIRECTION ( 'NONE',  ( 1.000000000000000000, 0.000000000000000000, 0.000000000000000000 ) ) ;
#7721=ORIENTED_EDGE ( 'NONE', *, *, #4041, .F. ) ;
#7729=LINE ( 'NONE', #8872, #160 ) ;
#7740=CARTESIAN_POINT ( 'NONE',  ( 88.84370878116858705, 10.64188714589527507, 2.999999999999999112 ) ) ;
#7759=CARTESIAN_POINT ( 'NONE',  ( 58.14665764790533586, -0.9105996816177498454, 3.000000000000000000 ) ) ;
#7768=CIRCLE ( 'NONE', #3109, 2.999999999999975131 ) ;
#7778=DIRECTION ( 'NONE',  ( -2.081668171172168513E-16, 1.000000000000000000, 0.000000000000000000 ) ) ;
#7805=ORIENTED_EDGE ( 'NONE', *, *, #9002, .F. ) ;
#7810=DIRECTION ( 'NONE',  ( -1.000000000000000000, 0.000000000000000000, 0.000000000000000000 ) ) ;
#7816=ORIENTED_EDGE ( 'NONE', *, *, #7033, .T. ) ;
#7818=VERTEX_POINT ( 'NONE', #13947 ) ;
#7822=CARTESIAN_POINT ( 'NONE',  ( 101.6227766016837819, -9.999999999999994671, -131.1575142076926852 ) ) ;
#7833=AXIS2_PLACEMENT_3D ( 'NONE', #8867, #4345, #13562 ) ;
#7840=DIRECTION ( 'NONE',  ( 1.000000000000000000, 0.000000000000000000, 0.000000000000000000 ) ) ;
#7847=CARTESIAN_POINT ( 'NONE',  ( 88.84370878116858705, 10.64188714589527507, 2.999999999999999112 ) ) ;
#7859=VERTEX_POINT ( 'NONE', #9792 ) ;
#7872=VERTEX_POINT ( 'NONE', #6328 ) ;
#7882=PLANE ( 'NONE',  #7833 ) ;
#7892=EDGE_CURVE ( 'NONE', #13731, #2441, #13849, .T. ) ;
#7904=DIRECTION ( 'NONE',  ( 0.000000000000000000, 0.000000000000000000, 1.000000000000000000 ) ) ;
#7905=EDGE_CURVE ( 'NONE', #7872, #5284, #7413, .T. ) ;
#7906=ORIENTED_EDGE ( 'NONE', *, *, #6296, .F. ) ;
#7937=ORIENTED_EDGE ( 'NONE', *, *, #1964, .F. ) ;
#7946=DIRECTION ( 'NONE',  ( 0.000000000000000000, 0.000000000000000000, -1.000000000000000000 ) ) ;
#8003=UNCERTAINTY_MEASURE_WITH_UNIT (LENGTH_MEASURE( 1.000000000000000082E-05 ), #961, 'distance_accuracy_value', 'NONE');
#8008=AXIS2_PLACEMENT_3D ( 'NONE', #13255, #12020, #9721 ) ;
#8010=DIRECTION ( 'NONE',  ( 1.000000000000000000, 0.000000000000000000, 0.000000000000000000 ) ) ;
#8013=DIRECTION ( 'NONE',  ( 0.000000000000000000, 0.000000000000000000, 1.000000000000000000 ) ) ;
#8021=ORIENTED_EDGE ( 'NONE', *, *, #4103, .F. ) ;
#8043=DIRECTION ( 'NONE',  ( 0.000000000000000000, 0.000000000000000000, 1.000000000000000000 ) ) ;
#8049=EDGE_CURVE ( 'NONE', #13244, #12675, #2020, .T. ) ;
#8067=PLANE ( 'NONE',  #794 ) ;
#8071=EDGE_CURVE ( 'NONE', #8563, #5508, #13086, .T. ) ;
#8092=DIRECTION ( 'NONE',  ( 1.000000000000000000, -6.245004513516508695E-15, 0.000000000000000000 ) ) ;
#8100=VERTEX_POINT ( 'NONE', #11981 ) ;
#8113=ORIENTED_EDGE ( 'NONE', *, *, #6452, .T. ) ;
#8131=CARTESIAN_POINT ( 'NONE',  ( 14.40394475573011945, -10.79473832354794460, 22.47056274847713908 ) ) ;
#8132=CARTESIAN_POINT ( 'NONE',  ( 33.82574562093736859, -6.697933970950280091, 2.999999999999999112 ) ) ;
#8135=DIRECTION ( 'NONE',  ( 0.000000000000000000, 0.000000000000000000, -1.000000000000000000 ) ) ;
#8136=DIRECTION ( 'NONE',  ( -0.000000000000000000, -0.000000000000000000, 1.000000000000000000 ) ) ;
#8139=FACE_OUTER_BOUND ( 'NONE', #2602, .T. ) ;
#8148=EDGE_CURVE ( 'NONE', #4678, #13200, #12119, .T. ) ;
#8159=EDGE_CURVE ( 'NONE', #15027, #108, #7396, .T. ) ;
#8179=ORIENTED_EDGE ( 'NONE', *, *, #12328, .T. ) ;
#8189=CYLINDRICAL_SURFACE ( 'NONE', #10034, 6.000000000000005329 ) ;
#8193=DIRECTION ( 'NONE',  ( -0.000000000000000000, -0.000000000000000000, 1.000000000000000000 ) ) ;
#8196=VECTOR ( 'NONE', #239, 999.9999999999998863 ) ;
#8199=DIRECTION ( 'NONE',  ( -0.000000000000000000, -0.000000000000000000, -1.000000000000000000 ) ) ;
#8206=VECTOR ( 'NONE', #4620, 1000.000000000000000 ) ;
#8213=EDGE_CURVE ( 'NONE', #12316, #15059, #2320, .T. ) ;
#8218=FACE_BOUND ( 'NONE', #12969, .T. ) ;
#8228=EDGE_CURVE ( 'NONE', #7557, #11633, #11148, .T. ) ;
#8239=EDGE_CURVE ( 'NONE', #11238, #4224, #2928, .T. ) ;
#8242=CARTESIAN_POINT ( 'NONE',  ( 80.82762530298222714, -19.99999999999999645, -131.1575142076926852 ) ) ;
#8249=DIRECTION ( 'NONE',  ( -0.000000000000000000, -0.000000000000000000, 1.000000000000000000 ) ) ;
#8264=VECTOR ( 'NONE', #2904, 1000.000000000000000 ) ;
#8278=CIRCLE ( 'NONE', #10253, 4.999999999999997335 ) ;
#8284=ORIENTED_EDGE ( 'NONE', *, *, #8413, .T. ) ;
#8299=FACE_BOUND ( 'NONE', #5038, .T. ) ;
#8303=EDGE_CURVE ( 'NONE', #3308, #3757, #913, .T. ) ;
#8306=AXIS2_PLACEMENT_3D ( 'NONE', #14752, #6602, #4516 ) ;
#8309=CARTESIAN_POINT ( 'NONE',  ( 98.63205416320636232, -2.094184955359725375, 6.000000000000000000 ) ) ;
#8357=FACE_BOUND ( 'NONE', #10378, .T. ) ;
#8363=DIRECTION ( 'NONE',  ( 0.000000000000000000, 0.000000000000000000, 1.000000000000000000 ) ) ;
#8392=ORIENTED_EDGE ( 'NONE', *, *, #5818, .F. ) ;
#8394=DIRECTION ( 'NONE',  ( 0.9988110320138940956, 0.04874958797097353469, 0.000000000000000000 ) ) ;
#8413=EDGE_CURVE ( 'NONE', #5313, #5535, #6180, .T. ) ;
#8437=VECTOR ( 'NONE', #12780, 1000.000000000000000 ) ;
#8440=ORIENTED_EDGE ( 'NONE', *, *, #3827, .T. ) ;
#8477=ORIENTED_EDGE ( 'NONE', *, *, #264, .F. ) ;
#8485=CIRCLE ( 'NONE', #12670, 2.999999999999988898 ) ;
#8490=CARTESIAN_POINT ( 'NONE',  ( 18.40394475573011945, -10.79473832354794460, 6.000000000000000000 ) ) ;
#8497=ORIENTED_EDGE ( 'NONE', *, *, #11881, .T. ) ;
#8512=EDGE_LOOP ( 'NONE', ( #3584, #5304, #5987, #13169 ) ) ;
#8516=CARTESIAN_POINT ( 'NONE',  ( 80.00000000000000000, 0.000000000000000000, 6.000000000000000000 ) ) ;
#8523=ORIENTED_EDGE ( 'NONE', *, *, #14307, .F. ) ;
#8535=CARTESIAN_POINT ( 'NONE',  ( 33.82574562093736859, -6.697933970950280091, 2.999999999999999112 ) ) ;
#8538=CARTESIAN_POINT ( 'NONE',  ( 80.00000000000000000, -9.999999999999994671, 6.000000000000000000 ) ) ;
#8552=EDGE_CURVE ( 'NONE', #4548, #3235, #6409, .T. ) ;
#8560=EDGE_LOOP ( 'NONE', ( #11746, #9943, #10702, #3646 ) ) ;
#8563=VERTEX_POINT ( 'NONE', #554 ) ;
#8579=VERTEX_POINT ( 'NONE', #5272 ) ;
#8594=DIRECTION ( 'NONE',  ( -1.000000000000000000, 0.000000000000000000, 0.000000000000000000 ) ) ;
#8602=EDGE_LOOP ( 'NONE', ( #2952, #5564, #8113, #2314 ) ) ;
#8610=DIRECTION ( 'NONE',  ( -0.000000000000000000, -0.000000000000000000, 1.000000000000000000 ) ) ;
#8634=ORIENTED_EDGE ( 'NONE', *, *, #460, .F. ) ;
#8636=CARTESIAN_POINT ( 'NONE',  ( 80.00000000000000000, 0.000000000000000000, 5.500000000000000000 ) ) ;
#8640=FACE_BOUND ( 'NONE', #123, .T. ) ;
#8643=DIRECTION ( 'NONE',  ( -0.9148936170212765839, -0.4036950204470272086, 0.000000000000000000 ) ) ;
#8648=ORIENTED_EDGE ( 'NONE', *, *, #8303, .T. ) ;
#8652=CARTESIAN_POINT ( 'NONE',  ( 101.6227766016837819, -9.999999999999994671, 3.000000000000002665 ) ) ;
#8715=CARTESIAN_POINT ( 'NONE',  ( 14.40394475573011945, -10.79473832354794460, 5.500000000000001776 ) ) ;
#8717=ORIENTED_EDGE ( 'NONE', *, *, #5625, .T. ) ;
#8720=AXIS2_PLACEMENT_3D ( 'NONE', #11008, #8778, #233 ) ;
#8722=EDGE_CURVE ( 'NONE', #13244, #8579, #7501, .T. ) ;
#8737=FACE_OUTER_BOUND ( 'NONE', #1788, .T. ) ;
#8749=FACE_OUTER_BOUND ( 'NONE', #1079, .T. ) ;
#8753=DIRECTION ( 'NONE',  ( -1.000000000000000000, 0.000000000000000000, 0.000000000000000000 ) ) ;
#8766=EDGE_LOOP ( 'NONE', ( #14875, #2672, #8021, #3773 ) ) ;
#8767=ORIENTED_EDGE ( 'NONE', *, *, #11437, .T. ) ;
#8778=DIRECTION ( 'NONE',  ( -0.000000000000000000, -0.000000000000000000, 1.000000000000000000 ) ) ;
#8783=AXIS2_PLACEMENT_3D ( 'NONE', #7312, #7079, #5932 ) ;
#8794=DIRECTION ( 'NONE',  ( -0.000000000000000000, -0.000000000000000000, -1.000000000000000000 ) ) ;
#8797=FACE_OUTER_BOUND ( 'NONE', #8766, .T. ) ;
#8805=ORIENTED_EDGE ( 'NONE', *, *, #11532, .T. ) ;
#8816=PLANE ( 'NONE',  #11752 ) ;
#8819=LINE ( 'NONE', #1453, #2903 ) ;
#8843=ORIENTED_EDGE ( 'NONE', *, *, #5331, .T. ) ;
#8853=CYLINDRICAL_SURFACE ( 'NONE', #1921, 10.00000000000000000 ) ;
#8859=CARTESIAN_POINT ( 'NONE',  ( 70.16198417812034904, 9.730076655429538590, 2.999999999999999112 ) ) ;
#8864=CARTESIAN_POINT ( 'NONE',  ( 98.63205416320636232, -2.094184955359750244, 3.000000000000000000 ) ) ;
#8867=CARTESIAN_POINT ( 'NONE',  ( 31.51081190520435626, 3.030430839836910639, 2.999999999999999112 ) ) ;
#8872=CARTESIAN_POINT ( 'NONE',  ( 58.14665764790533586, -0.9105996816177489572, 2.999999999999999112 ) ) ;
#8894=CARTESIAN_POINT ( 'NONE',  ( -5.999999999999999112, 0.000000000000000000, 5.500000000000000000 ) ) ;
#8911=EDGE_CURVE ( 'NONE', #15059, #12037, #7628, .T. ) ;
#8918=EDGE_CURVE ( 'NONE', #12675, #5309, #9695, .T. ) ;
#8942=LINE ( 'NONE', #13719, #11417 ) ;
#8969=PLANE ( 'NONE',  #8306 ) ;
#8990=CIRCLE ( 'NONE', #11442, 4.000000000000000000 ) ;
#8993=VECTOR ( 'NONE', #3714, 1000.000000000000000 ) ;
#9002=EDGE_CURVE ( 'NONE', #9526, #7097, #11901, .T. ) ;
#9006=VECTOR ( 'NONE', #6230, 1000.000000000000114 ) ;
#9019=VERTEX_POINT ( 'NONE', #13998 ) ;
#9036=AXIS2_PLACEMENT_3D ( 'NONE', #12806, #10592, #5840 ) ;
#9049=CARTESIAN_POINT ( 'NONE',  ( 10.40394475573011945, -10.79473832354794460, 5.500000000000000000 ) ) ;
#9052=DIRECTION ( 'NONE',  ( 0.8893705212896308998, -0.4571871344001384729, 0.000000000000000000 ) ) ;
#9080=ORIENTED_EDGE ( 'NONE', *, *, #9480, .F. ) ;
#9094=VECTOR ( 'NONE', #15124, 1000.000000000000000 ) ;
#9103=ORIENTED_EDGE ( 'NONE', *, *, #1044, .F. ) ;
#9104=( NAMED_UNIT ( * ) PLANE_ANGLE_UNIT ( ) SI_UNIT ( $, .RADIAN. ) );
#9116=DIRECTION ( 'NONE',  ( 0.5416238976136762417, -0.8406209333187997235, 0.000000000000000000 ) ) ;
#9152=VECTOR ( 'NONE', #1518, 1000.000000000000000 ) ;
#9158=DIRECTION ( 'NONE',  ( 0.1643989873053573469, -0.9863939238321437486, 0.000000000000000000 ) ) ;
#9161=EDGE_CURVE ( 'NONE', #214, #3838, #14672, .T. ) ;
#9164=DIRECTION ( 'NONE',  ( -0.4571871344001416926, -0.8893705212896291235, -0.000000000000000000 ) ) ;
#9182=DIRECTION ( 'NONE',  ( -0.000000000000000000, -0.000000000000000000, 1.000000000000000000 ) ) ;
#9195=LINE ( 'NONE', #10273, #12467 ) ;
#9212=ORIENTED_EDGE ( 'NONE', *, *, #2721, .T. ) ;
#9228=VERTEX_POINT ( 'NONE', #3996 ) ;
#9266=FACE_OUTER_BOUND ( 'NONE', #5255, .T. ) ;
#9281=LINE ( 'NONE', #10424, #9094 ) ;
#9283=CARTESIAN_POINT ( 'NONE',  ( 80.00000000000000000, 0.000000000000000000, 5.500000000000000000 ) ) ;
#9284=CARTESIAN_POINT ( 'NONE',  ( 80.00000000000000000, 0.000000000000000000, 5.500000000000000000 ) ) ;
#9290=LINE ( 'NONE', #246, #8993 ) ;
#9301=CARTESIAN_POINT ( 'NONE',  ( 0.000000000000000000, 0.000000000000000000, 5.500000000000000000 ) ) ;
#9314=ORIENTED_EDGE ( 'NONE', *, *, #5178, .T. ) ;
#9343=CARTESIAN_POINT ( 'NONE',  ( 67.45386469005195806, 13.93318132202354676, 2.999999999999999112 ) ) ;
#9364=EDGE_CURVE ( 'NONE', #677, #14436, #6224, .T. ) ;
#9374=ORIENTED_EDGE ( 'NONE', *, *, #11437, .F. ) ;
#9382=ORIENTED_EDGE ( 'NONE', *, *, #13311, .F. ) ;
#9383=DIRECTION ( 'NONE',  ( 1.000000000000000000, 0.000000000000000000, 0.000000000000000000 ) ) ;
#9385=CIRCLE ( 'NONE', #2522, 3.000000000000002665 ) ;
#9398=DIRECTION ( 'NONE',  ( 1.000000000000000000, 0.000000000000000000, 0.000000000000000000 ) ) ;
#9411=CARTESIAN_POINT ( 'NONE',  ( -9.999999999999998224, -1.390791565672605534, 6.000000000000000000 ) ) ;
#9419=ORIENTED_EDGE ( 'NONE', *, *, #8911, .F. ) ;
#9427=DIRECTION ( 'NONE',  ( -1.000000000000000000, 0.000000000000000000, 0.000000000000000000 ) ) ;
#9431=DIRECTION ( 'NONE',  ( -0.000000000000000000, -0.000000000000000000, 1.000000000000000000 ) ) ;
#9433=LINE ( 'NONE', #14129, #2458 ) ;
#9436=ORIENTED_EDGE ( 'NONE', *, *, #4867, .F. ) ;
#9439=AXIS2_PLACEMENT_3D ( 'NONE', #5094, #9769, #454 ) ;
#9450=CARTESIAN_POINT ( 'NONE',  ( 80.00000000000000000, 0.000000000000000000, 5.500000000000005329 ) ) ;
#9457=AXIS2_PLACEMENT_3D ( 'NONE', #4427, #6872, #2410 ) ;
#9461=ORIENTED_EDGE ( 'NONE', *, *, #4325, .F. ) ;
#9465=ORIENTED_EDGE ( 'NONE', *, *, #8049, .F. ) ;
#9480=EDGE_CURVE ( 'NONE', #5284, #6485, #5371, .T. ) ;
#9497=CARTESIAN_POINT ( 'NONE',  ( 0.000000000000000000, 0.000000000000000000, 6.000000000000000000 ) ) ;
#9505=MECHANICAL_DESIGN_GEOMETRIC_PRESENTATION_REPRESENTATION('',(#7551),#1163);
#9521=CARTESIAN_POINT ( 'NONE',  ( 1.666666666666673624, 0.000000000000000000, -131.1575142076926852 ) ) ;
#9523=AXIS2_PLACEMENT_3D ( 'NONE', #13079, #13252, #10798 ) ;
#9526=VERTEX_POINT ( 'NONE', #7057 ) ;
#9527=AXIS2_PLACEMENT_3D ( 'NONE', #14367, #9829, #6289 ) ;
#9541=EDGE_CURVE ( 'NONE', #5309, #12675, #2161, .T. ) ;
#9564=EDGE_LOOP ( 'NONE', ( #14661, #7721, #9374, #14120 ) ) ;
#9586=CARTESIAN_POINT ( 'NONE',  ( 88.84370878116858705, 10.64188714589527507, 2.999999999999999112 ) ) ;
#9592=EDGE_LOOP ( 'NONE', ( #9103, #5169, #3295, #4398 ) ) ;
#9593=DIRECTION ( 'NONE',  ( 0.000000000000000000, 0.000000000000000000, 1.000000000000000000 ) ) ;
#9599=VERTEX_POINT ( 'NONE', #13105 ) ;
#9607=CARTESIAN_POINT ( 'NONE',  ( 93.34550147531103903, 3.654933296868752457, 2.999999999999999112 ) ) ;
#9617=ORIENTED_EDGE ( 'NONE', *, *, #11882, .T. ) ;
#9620=DIRECTION ( 'NONE',  ( 0.000000000000000000, 0.000000000000000000, 1.000000000000000000 ) ) ;
#9625=EDGE_CURVE ( 'NONE', #5508, #14446, #1280, .T. ) ;
#9631=DIRECTION ( 'NONE',  ( 0.9148936170212765839, 0.4036950204470272086, -0.000000000000000000 ) ) ;
#9640=DIRECTION ( 'NONE',  ( 1.000000000000000000, 0.000000000000000000, 0.000000000000000000 ) ) ;
#9642=DIRECTION ( 'NONE',  ( -0.000000000000000000, -0.000000000000000000, -1.000000000000000000 ) ) ;
#9643=DIRECTION ( 'NONE',  ( -0.9988110320138940956, -0.04874958797097371510, 0.000000000000000000 ) ) ;
#9664=ORIENTED_EDGE ( 'NONE', *, *, #8148, .T. ) ;
#9667=CLOSED_SHELL ( 'NONE', ( #3976, #12651, #1992, #4037, #11219, #1981, #7335, #11684, #7165, #14805, #7109, #6650, #13335, #11367, #13288, #7685, #14155, #10413, #13324, #7428, #6933, #2856, #6523, #14515, #6854, #13295, #14065, #10166, #7199, #13480, #6276, #11254, #234, #14078, #6622, #1407, #4851, #11707, #97, #11787, #9831, #11701, #6433, #12380, #746, #4545, #13615 ) ) ;
#9676=ORIENTED_EDGE ( 'NONE', *, *, #3440, .T. ) ;
#9686=EDGE_CURVE ( 'NONE', #108, #7872, #8278, .T. ) ;
#9692=DIRECTION ( 'NONE',  ( 0.000000000000000000, 0.000000000000000000, 1.000000000000000000 ) ) ;
#9695=CIRCLE ( 'NONE', #3079, 4.000000000000000000 ) ;
#9721=DIRECTION ( 'NONE',  ( 1.000000000000000000, 0.000000000000000000, 0.000000000000000000 ) ) ;
#9731=VERTEX_POINT ( 'NONE', #6279 ) ;
#9739=AXIS2_PLACEMENT_3D ( 'NONE', #14062, #861, #14297 ) ;
#9761=VERTEX_POINT ( 'NONE', #8652 ) ;
#9769=DIRECTION ( 'NONE',  ( 0.000000000000000000, 0.000000000000000000, -1.000000000000000000 ) ) ;
#9771=AXIS2_PLACEMENT_3D ( 'NONE', #8636, #11096, #7264 ) ;
#9772=DIRECTION ( 'NONE',  ( -1.000000000000000000, 0.000000000000000000, 0.000000000000000000 ) ) ;
#9792=CARTESIAN_POINT ( 'NONE',  ( 91.46153288930040048, 16.46030115554384565, 2.999999999999999112 ) ) ;
#9805=CARTESIAN_POINT ( 'NONE',  ( 80.82762530298222714, -19.99999999999999645, 3.000000000000002665 ) ) ;
#9829=DIRECTION ( 'NONE',  ( 0.000000000000000000, 0.000000000000000000, 1.000000000000000000 ) ) ;
#9831=ADVANCED_FACE ( 'NONE', ( #12641 ), #4439, .F. ) ;
#9855=CYLINDRICAL_SURFACE ( 'NONE', #14388, 4.000000000000003553 ) ;
#9863=ORIENTED_EDGE ( 'NONE', *, *, #6293, .F. ) ;
#9868=FACE_OUTER_BOUND ( 'NONE', #11489, .T. ) ;
#9878=AXIS2_PLACEMENT_3D ( 'NONE', #10444, #9431, #6981 ) ;
#9902=CYLINDRICAL_SURFACE ( 'NONE', #6551, 4.000000000000003553 ) ;
#9904=CARTESIAN_POINT ( 'NONE',  ( 88.84370878116860126, 10.64188714589527684, 6.000000000000000000 ) ) ;
#9906=DIRECTION ( 'NONE',  ( -0.000000000000000000, -0.000000000000000000, -1.000000000000000000 ) ) ;
#9927=FACE_OUTER_BOUND ( 'NONE', #13333, .T. ) ;
#9931=VECTOR ( 'NONE', #8043, 1000.000000000000000 ) ;
#9933=VECTOR ( 'NONE', #4181, 1000.000000000000114 ) ;
#9943=ORIENTED_EDGE ( 'NONE', *, *, #6507, .T. ) ;
#9960=CIRCLE ( 'NONE', #3333, 2.999999999999988898 ) ;
#9962=ORIENTED_EDGE ( 'NONE', *, *, #340, .T. ) ;
#9964=ORIENTED_EDGE ( 'NONE', *, *, #6159, .T. ) ;
#9976=DIRECTION ( 'NONE',  ( -0.000000000000000000, -0.000000000000000000, -1.000000000000000000 ) ) ;
#9984=AXIS2_PLACEMENT_3D ( 'NONE', #12157, #1643, #8394 ) ;
#9992=CIRCLE ( 'NONE', #7034, 3.000000000000002665 ) ;
#10024=DIRECTION ( 'NONE',  ( 1.000000000000000000, 0.000000000000000000, 0.000000000000000000 ) ) ;
#10032=CARTESIAN_POINT ( 'NONE',  ( 5.999999999999999112, 7.347880794884118750E-16, 3.000000000000000000 ) ) ;
#10034=AXIS2_PLACEMENT_3D ( 'NONE', #9283, #7045, #10582 ) ;
#10039=( NAMED_UNIT ( * ) SI_UNIT ( $, .STERADIAN. ) SOLID_ANGLE_UNIT ( ) );
#10064=ORIENTED_EDGE ( 'NONE', *, *, #4223, .F. ) ;
#10083=DIRECTION ( 'NONE',  ( 0.000000000000000000, 0.000000000000000000, -1.000000000000000000 ) ) ;
#10085=CARTESIAN_POINT ( 'NONE',  ( -4.000000000000000000, 0.000000000000000000, 5.500000000000000000 ) ) ;
#10089=DIRECTION ( 'NONE',  ( -0.000000000000000000, -0.000000000000000000, 1.000000000000000000 ) ) ;
#10105=ORIENTED_EDGE ( 'NONE', *, *, #2970, .F. ) ;
#10110=EDGE_CURVE ( 'NONE', #3838, #4613, #1425, .T. ) ;
#10121=DIRECTION ( 'NONE',  ( 0.000000000000000000, 0.000000000000000000, 1.000000000000000000 ) ) ;
#10134=CARTESIAN_POINT ( 'NONE',  ( 13.28797974610714761, -21.11867004231547540, 3.000000000000002665 ) ) ;
#10160=ORIENTED_EDGE ( 'NONE', *, *, #10286, .F. ) ;
#10161=CYLINDRICAL_SURFACE ( 'NONE', #15100, 2.999999999999975131 ) ;
#10166=ADVANCED_FACE ( 'NONE', ( #14332 ), #487, .F. ) ;
#10168=AXIS2_PLACEMENT_3D ( 'NONE', #14617, #14322, #12371 ) ;
#10173=ORIENTED_EDGE ( 'NONE', *, *, #1384, .T. ) ;
#10184=DIRECTION ( 'NONE',  ( 0.000000000000000000, 0.000000000000000000, 1.000000000000000000 ) ) ;
#10222=AXIS2_PLACEMENT_3D ( 'NONE', #10533, #8193, #4701 ) ;
#10224=AXIS2_PLACEMENT_3D ( 'NONE', #981, #2060, #679 ) ;
#10233=EDGE_CURVE ( 'NONE', #6410, #14061, #11971, .T. ) ;
#10243=CARTESIAN_POINT ( 'NONE',  ( 14.40394475573011945, -10.79473832354794460, 6.000000000000000000 ) ) ;
#10244=DIRECTION ( 'NONE',  ( 0.000000000000000000, 0.000000000000000000, 1.000000000000000000 ) ) ;
#10250=MECHANICAL_DESIGN_GEOMETRIC_PRESENTATION_REPRESENTATION('',(#1915),#3873);
#10253=AXIS2_PLACEMENT_3D ( 'NONE', #6506, #664, #2678 ) ;
#10255=EDGE_LOOP ( 'NONE', ( #11562, #9436, #18, #9212 ) ) ;
#10257=( LENGTH_UNIT ( ) NAMED_UNIT ( * ) SI_UNIT ( .MILLI., .METRE. ) );
#10273=CARTESIAN_POINT ( 'NONE',  ( 61.98919079003883326, 3.953582723775848962, 2.999999999999999112 ) ) ;
#10277=DIRECTION ( 'NONE',  ( -1.000000000000000000, 0.000000000000000000, 0.000000000000000000 ) ) ;
#10279=VERTEX_POINT ( 'NONE', #5863 ) ;
#10282=LINE ( 'NONE', #8894, #534 ) ;
#10286=EDGE_CURVE ( 'NONE', #11305, #12316, #11251, .T. ) ;
#10294=EDGE_LOOP ( 'NONE', ( #4259, #1494, #4481, #8440 ) ) ;
#10302=ORIENTED_EDGE ( 'NONE', *, *, #4714, .T. ) ;
#10305=ORIENTED_EDGE ( 'NONE', *, *, #4604, .T. ) ;
#10313=CARTESIAN_POINT ( 'NONE',  ( 20.40394475573011590, -10.79473832354794460, 3.000000000000000000 ) ) ;
#10335=CARTESIAN_POINT ( 'NONE',  ( 10.00000000000000178, -1.390791565672601315, -131.1575142076926852 ) ) ;
#10337=CARTESIAN_POINT ( 'NONE',  ( 31.51081190520435626, 3.030430839836910639, 6.000000000000000000 ) ) ;
#10351=CIRCLE ( 'NONE', #5944, 6.000000000000005329 ) ;
#10354=CARTESIAN_POINT ( 'NONE',  ( 88.46153288930041469, 16.46030115554384565, 6.000000000000000000 ) ) ;
#10378=EDGE_LOOP ( 'NONE', ( #10305, #13834 ) ) ;
#10386=CYLINDRICAL_SURFACE ( 'NONE', #1419, 11.66666666666667318 ) ;
#10395=EDGE_CURVE ( 'NONE', #5489, #9019, #7229, .T. ) ;
#10400=CARTESIAN_POINT ( 'NONE',  ( 61.98919079003883326, 3.953582723775848962, 6.000000000000000000 ) ) ;
#10413=ADVANCED_FACE ( 'NONE', ( #10767 ), #12899, .T. ) ;
#10417=AXIS2_PLACEMENT_3D ( 'NONE', #1539, #9906, #12056 ) ;
#10424=CARTESIAN_POINT ( 'NONE',  ( 80.82762530298222714, -9.999999999999994671, 3.000000000000002665 ) ) ;
#10444=CARTESIAN_POINT ( 'NONE',  ( 14.40394475573011945, -10.79473832354794460, 5.500000000000000000 ) ) ;
#10460=DIRECTION ( 'NONE',  ( 1.000000000000000000, 0.000000000000000000, 0.000000000000000000 ) ) ;
#10462=DIRECTION ( 'NONE',  ( -1.000000000000000000, 0.000000000000000000, 0.000000000000000000 ) ) ;
#10466=AXIS2_PLACEMENT_3D ( 'NONE', #5393, #14759, #2288 ) ;
#10467=ORIENTED_EDGE ( 'NONE', *, *, #7905, .F. ) ;
#10489=CARTESIAN_POINT ( 'NONE',  ( 91.46153288930040048, 16.46030115554384565, 2.999999999999999112 ) ) ;
#10505=CYLINDRICAL_SURFACE ( 'NONE', #864, 3.000000000000002665 ) ;
#10509=DIRECTION ( 'NONE',  ( 0.000000000000000000, 0.000000000000000000, 1.000000000000000000 ) ) ;
#10513=CARTESIAN_POINT ( 'NONE',  ( 88.46153288930041469, 16.46030115554384565, 2.999999999999999112 ) ) ;
#10524=FACE_OUTER_BOUND ( 'NONE', #11757, .T. ) ;
#10533=CARTESIAN_POINT ( 'NONE',  ( 72.68384697807672978, 11.35494834827056110, 2.999999999999999112 ) ) ;
#10554=DIRECTION ( 'NONE',  ( 1.000000000000000000, 0.000000000000000000, 0.000000000000000000 ) ) ;
#10556=ORIENTED_EDGE ( 'NONE', *, *, #11882, .F. ) ;
#10562=CARTESIAN_POINT ( 'NONE',  ( 5.999999999999999112, 7.347880794884118750E-16, 5.500000000000000000 ) ) ;
#10572=EDGE_LOOP ( 'NONE', ( #788, #13664, #562, #7051 ) ) ;
#10582=DIRECTION ( 'NONE',  ( -1.000000000000000000, 0.000000000000000000, 0.000000000000000000 ) ) ;
#10591=CYLINDRICAL_SURFACE ( 'NONE', #14422, 6.000000000000000000 ) ;
#10592=DIRECTION ( 'NONE',  ( 0.000000000000000000, 0.000000000000000000, 1.000000000000000000 ) ) ;
#10601=VERTEX_POINT ( 'NONE', #2225 ) ;
#10608=DIRECTION ( 'NONE',  ( 1.000000000000000000, 0.000000000000000000, 0.000000000000000000 ) ) ;
#10612=DIRECTION ( 'NONE',  ( 0.000000000000000000, -0.000000000000000000, -1.000000000000000000 ) ) ;
#10634=DIRECTION ( 'NONE',  ( -1.000000000000000000, 0.000000000000000000, 0.000000000000000000 ) ) ;
#10655=AXIS2_PLACEMENT_3D ( 'NONE', #3023, #13705, #7708 ) ;
#10664=ORIENTED_EDGE ( 'NONE', *, *, #2429, .F. ) ;
#10669=EDGE_LOOP ( 'NONE', ( #2752, #14315, #1659, #14773 ) ) ;
#10670=FACE_OUTER_BOUND ( 'NONE', #11596, .T. ) ;
#10682=FACE_BOUND ( 'NONE', #11318, .T. ) ;
#10689=DIRECTION ( 'NONE',  ( 0.000000000000000000, 0.000000000000000000, -1.000000000000000000 ) ) ;
#10699=PRODUCT ( 'plate 2', 'plate 2', '', ( #666 ) ) ;
#10701=EDGE_CURVE ( 'NONE', #12700, #6090, #13755, .T. ) ;
#10702=ORIENTED_EDGE ( 'NONE', *, *, #10233, .T. ) ;
#10717=VECTOR ( 'NONE', #9631, 1000.000000000000114 ) ;
#10726=DIRECTION ( 'NONE',  ( 0.000000000000000000, 0.000000000000000000, -1.000000000000000000 ) ) ;
#10742=EDGE_CURVE ( 'NONE', #11509, #1482, #4462, .T. ) ;
#10752=CARTESIAN_POINT ( 'NONE',  ( 85.79342132543153809, 17.83186255874426962, 2.999999999999999112 ) ) ;
#10753=DIRECTION ( 'NONE',  ( -0.000000000000000000, -0.000000000000000000, -1.000000000000000000 ) ) ;
#10767=FACE_OUTER_BOUND ( 'NONE', #5129, .T. ) ;
#10782=CYLINDRICAL_SURFACE ( 'NONE', #8720, 2.999999999999988898 ) ;
#10785=CARTESIAN_POINT ( 'NONE',  ( 20.40394475573011590, -10.79473832354794460, 5.500000000000001776 ) ) ;
#10792=DIRECTION ( 'NONE',  ( -0.9728364810787193395, -0.2314933715733012709, -0.000000000000000000 ) ) ;
#10798=DIRECTION ( 'NONE',  ( 1.000000000000000000, 0.000000000000000000, 0.000000000000000000 ) ) ;
#10823=CYLINDRICAL_SURFACE ( 'NONE', #1429, 4.000000000000000000 ) ;
#10830=EDGE_LOOP ( 'NONE', ( #36, #11446 ) ) ;
#10836=CARTESIAN_POINT ( 'NONE',  ( 0.000000000000000000, 0.000000000000000000, 5.500000000000000000 ) ) ;
#10843=CIRCLE ( 'NONE', #13041, 6.000000000000000000 ) ;
#10865=ORIENTED_EDGE ( 'NONE', *, *, #2481, .F. ) ;
#10871=LINE ( 'NONE', #14264, #14473 ) ;
#10872=LINE ( 'NONE', #6265, #13226 ) ;
#10873=ORIENTED_EDGE ( 'NONE', *, *, #7437, .T. ) ;
#10894=ORIENTED_EDGE ( 'NONE', *, *, #1571, .F. ) ;
#10920=DIRECTION ( 'NONE',  ( 1.000000000000000000, 0.000000000000000000, 0.000000000000000000 ) ) ;
#10924=AXIS2_PLACEMENT_3D ( 'NONE', #12326, #1803, #6488 ) ;
#10934=CARTESIAN_POINT ( 'NONE',  ( 98.48580539929344013, 0.9022481406819604643, 2.999999999999999112 ) ) ;
#10935=AXIS2_PLACEMENT_3D ( 'NONE', #13617, #5343, #4179 ) ;
#10944=VECTOR ( 'NONE', #2706, 1000.000000000000000 ) ;
#10958=ORIENTED_EDGE ( 'NONE', *, *, #2721, .F. ) ;
#10974=CARTESIAN_POINT ( 'NONE',  ( 79.18363542992865689, -10.13606076167855541, 3.000000000000002665 ) ) ;
#10984=EDGE_LOOP ( 'NONE', ( #5008, #10160, #5000, #5776 ) ) ;
#11007=UNCERTAINTY_MEASURE_WITH_UNIT (LENGTH_MEASURE( 1.000000000000000082E-05 ), #253, 'distance_accuracy_value', 'NONE');
#11008=CARTESIAN_POINT ( 'NONE',  ( 72.68384697807672978, 11.35494834827056110, 2.999999999999999112 ) ) ;
#11024=DIRECTION ( 'NONE',  ( -0.000000000000000000, -0.000000000000000000, -1.000000000000000000 ) ) ;
#11040=CARTESIAN_POINT ( 'NONE',  ( 67.23404255319145761, 28.93147646537026318, 3.000000000000002665 ) ) ;
#11048=CARTESIAN_POINT ( 'NONE',  ( 86.00000000000000000, 7.347880794884121708E-16, 5.500000000000000000 ) ) ;
#11078=EDGE_CURVE ( 'NONE', #9761, #2630, #13652, .T. ) ;
#11080=ORIENTED_EDGE ( 'NONE', *, *, #7905, .T. ) ;
#11091=ORIENTED_EDGE ( 'NONE', *, *, #12490, .T. ) ;
#11092=DIRECTION ( 'NONE',  ( 1.000000000000000000, 0.000000000000000000, 0.000000000000000000 ) ) ;
#11096=DIRECTION ( 'NONE',  ( -0.000000000000000000, -0.000000000000000000, -1.000000000000000000 ) ) ;
#11099=DIRECTION ( 'NONE',  ( 1.000000000000000000, 0.000000000000000000, 0.000000000000000000 ) ) ;
#11122=LINE ( 'NONE', #445, #4327 ) ;
#11133=VERTEX_POINT ( 'NONE', #9049 ) ;
#11137=CARTESIAN_POINT ( 'NONE',  ( 98.33955663538051795, 3.898681236723621879, 6.000000000000000000 ) ) ;
#11141=EDGE_CURVE ( 'NONE', #2895, #5216, #11886, .T. ) ;
#11142=ORIENTED_EDGE ( 'NONE', *, *, #6450, .F. ) ;
#11144=EDGE_LOOP ( 'NONE', ( #6610, #6806, #8179, #5777 ) ) ;
#11148=CIRCLE ( 'NONE', #9439, 4.000000000000000000 ) ;
#11154=CARTESIAN_POINT ( 'NONE',  ( 59.05334708265790056, 38.04890259842303379, 6.000000000000000000 ) ) ;
#11172=DIRECTION ( 'NONE',  ( 0.000000000000000000, 0.000000000000000000, -1.000000000000000000 ) ) ;
#11176=SHAPE_REPRESENTATION_RELATIONSHIP ( 'NONE' , 'NONE' ,  #2588, #15172 ) ;
#11185=ORIENTED_EDGE ( 'NONE', *, *, #2329, .T. ) ;
#11190=CARTESIAN_POINT ( 'NONE',  ( 14.40394475573011945, -10.79473832354794460, 6.000000000000000000 ) ) ;
#11202=VECTOR ( 'NONE', #7320, 1000.000000000000000 ) ;
#11204=AXIS2_PLACEMENT_3D ( 'NONE', #1725, #6408, #11092 ) ;
#11206=CYLINDRICAL_SURFACE ( 'NONE', #10466, 4.999999999999997335 ) ;
#11218=DIRECTION ( 'NONE',  ( -0.000000000000000000, -0.000000000000000000, 1.000000000000000000 ) ) ;
#11219=ADVANCED_FACE ( 'NONE', ( #14029 ), #10505, .F. ) ;
#11238=VERTEX_POINT ( 'NONE', #4740 ) ;
#11243=LINE ( 'NONE', #4333, #6915 ) ;
#11244=AXIS2_PLACEMENT_3D ( 'NONE', #4115, #8794, #2959 ) ;
#11251=LINE ( 'NONE', #4555, #13454 ) ;
#11254=ADVANCED_FACE ( 'NONE', ( #7188 ), #7116, .F. ) ;
#11259=AXIS2_PLACEMENT_3D ( 'NONE', #12023, #1502, #332 ) ;
#11273=LINE ( 'NONE', #747, #6313 ) ;
#11276=DIRECTION ( 'NONE',  ( 1.000000000000000000, 0.000000000000000000, 0.000000000000000000 ) ) ;
#11279=EDGE_LOOP ( 'NONE', ( #1693, #2286, #4187, #12765 ) ) ;
#11305=VERTEX_POINT ( 'NONE', #5363 ) ;
#11306=EDGE_LOOP ( 'NONE', ( #9419, #14108, #2330, #8477 ) ) ;
#11309=CARTESIAN_POINT ( 'NONE',  ( 0.000000000000000000, 0.000000000000000000, 5.500000000000000000 ) ) ;
#11310=EDGE_CURVE ( 'NONE', #6202, #3359, #12402, .T. ) ;
#11318=EDGE_LOOP ( 'NONE', ( #193, #5515 ) ) ;
#11360=ORIENTED_EDGE ( 'NONE', *, *, #3329, .T. ) ;
#11367=ADVANCED_FACE ( 'NONE', ( #2960, #7577, #13406, #8640, #14419, #7648, #13256, #3887 ), #12092, .T. ) ;
#11382=VECTOR ( 'NONE', #7409, 1000.000000000000000 ) ;
#11399=FACE_OUTER_BOUND ( 'NONE', #11306, .T. ) ;
#11417=VECTOR ( 'NONE', #11551, 1000.000000000000114 ) ;
#11437=EDGE_CURVE ( 'NONE', #10601, #5949, #8942, .T. ) ;
#11442=AXIS2_PLACEMENT_3D ( 'NONE', #5325, #13532, #3003 ) ;
#11444=AXIS2_PLACEMENT_3D ( 'NONE', #10934, #12802, #3880 ) ;
#11446=ORIENTED_EDGE ( 'NONE', *, *, #8228, .T. ) ;
#11462=EDGE_LOOP ( 'NONE', ( #4245, #11185, #4087, #14250 ) ) ;
#11471=CARTESIAN_POINT ( 'NONE',  ( 4.000000000000000000, 4.898587196589412829E-16, 5.500000000000000000 ) ) ;
#11477=CARTESIAN_POINT ( 'NONE',  ( 10.00000000000000178, -1.390791565672601315, 6.000000000000005329 ) ) ;
#11478=EDGE_LOOP ( 'NONE', ( #7475, #14474 ) ) ;
#11489=EDGE_LOOP ( 'NONE', ( #979, #14567, #12679, #1364 ) ) ;
#11497=EDGE_CURVE ( 'NONE', #6090, #11305, #13374, .T. ) ;
#11502=CARTESIAN_POINT ( 'NONE',  ( 93.49175023922396122, 0.6585002008270834928, 6.000000000000000000 ) ) ;
#11509=VERTEX_POINT ( 'NONE', #8864 ) ;
#11517=CARTESIAN_POINT ( 'NONE',  ( 72.68384697807672978, 11.35494834827056110, 2.999999999999999112 ) ) ;
#11521=CARTESIAN_POINT ( 'NONE',  ( 93.63799900313688340, -2.337932895214618778, 6.000000000000000000 ) ) ;
#11530=EDGE_CURVE ( 'NONE', #4613, #4354, #12149, .T. ) ;
#11532=EDGE_CURVE ( 'NONE', #7859, #6954, #1114, .T. ) ;
#11537=ORIENTED_EDGE ( 'NONE', *, *, #4868, .T. ) ;
#11538=DIRECTION ( 'NONE',  ( 0.000000000000000000, 0.000000000000000000, -1.000000000000000000 ) ) ;
#11541=DIRECTION ( 'NONE',  ( 0.000000000000000000, 0.000000000000000000, 1.000000000000000000 ) ) ;
#11551=DIRECTION ( 'NONE',  ( -0.5416238976136773520, 0.8406209333187989463, 0.000000000000000000 ) ) ;
#11562=ORIENTED_EDGE ( 'NONE', *, *, #6507, .F. ) ;
#11583=FACE_OUTER_BOUND ( 'NONE', #6047, .T. ) ;
#11596=EDGE_LOOP ( 'NONE', ( #3093, #5591, #466, #1041 ) ) ;
#11608=DIRECTION ( 'NONE',  ( -0.000000000000000000, -0.000000000000000000, 1.000000000000000000 ) ) ;
#11624=DIRECTION ( 'NONE',  ( -1.000000000000000000, -2.081668171172168513E-16, 0.000000000000000000 ) ) ;
#11625=LINE ( 'NONE', #10489, #578 ) ;
#11629=CYLINDRICAL_SURFACE ( 'NONE', #6210, 2.999999999999975131 ) ;
#11630=VECTOR ( 'NONE', #3676, 1000.000000000000227 ) ;
#11631=ORIENTED_EDGE ( 'NONE', *, *, #11310, .F. ) ;
#11633=VERTEX_POINT ( 'NONE', #1250 ) ;
#11640=CARTESIAN_POINT ( 'NONE',  ( 80.00000000000000000, 0.000000000000000000, 3.000000000000000000 ) ) ;
#11646=DIRECTION ( 'NONE',  ( 0.000000000000000000, 0.000000000000000000, -1.000000000000000000 ) ) ;
#11665=DIRECTION ( 'NONE',  ( -1.000000000000000000, 0.000000000000000000, 0.000000000000000000 ) ) ;
#11675=FACE_BOUND ( 'NONE', #7414, .T. ) ;
#11684=ADVANCED_FACE ( 'NONE', ( #310 ), #9855, .F. ) ;
#11701=ADVANCED_FACE ( 'NONE', ( #14553 ), #12148, .F. ) ;
#11705=DIRECTION ( 'NONE',  ( 1.000000000000000000, 0.000000000000000000, 0.000000000000000000 ) ) ;
#11707=ADVANCED_FACE ( 'NONE', ( #3947 ), #10782, .F. ) ;
#11709=EDGE_LOOP ( 'NONE', ( #14454, #4875 ) ) ;
#11714=AXIS2_PLACEMENT_3D ( 'NONE', #1800, #9158, #6778 ) ;
#11744=LINE ( 'NONE', #14212, #11630 ) ;
#11746=ORIENTED_EDGE ( 'NONE', *, *, #10395, .F. ) ;
#11752=AXIS2_PLACEMENT_3D ( 'NONE', #7740, #9052, #12425 ) ;
#11757=EDGE_LOOP ( 'NONE', ( #5021, #7696, #6288, #9664 ) ) ;
#11765=CARTESIAN_POINT ( 'NONE',  ( 8.403944755730119454, -10.79473832354794460, 22.47056274847713908 ) ) ;
#11787=ADVANCED_FACE ( 'NONE', ( #9927 ), #1865, .F. ) ;
#11789=CARTESIAN_POINT ( 'NONE',  ( 98.48580539929344013, 0.9022481406819604643, 2.999999999999999112 ) ) ;
#11792=ORIENTED_EDGE ( 'NONE', *, *, #8918, .F. ) ;
#11795=DIRECTION ( 'NONE',  ( 0.000000000000000000, 0.000000000000000000, -1.000000000000000000 ) ) ;
#11808=CARTESIAN_POINT ( 'NONE',  ( 70.16198417812034904, 9.730076655429538590, 2.999999999999999112 ) ) ;
#11810=LINE ( 'NONE', #7523, #3937 ) ;
#11821=ORIENTED_EDGE ( 'NONE', *, *, #1384, .F. ) ;
#11824=DIRECTION ( 'NONE',  ( 0.000000000000000000, 0.000000000000000000, 1.000000000000000000 ) ) ;
#11837=ORIENTED_EDGE ( 'NONE', *, *, #3073, .F. ) ;
#11844=DIRECTION ( 'NONE',  ( -0.000000000000000000, -0.000000000000000000, 1.000000000000000000 ) ) ;
#11872=VECTOR ( 'NONE', #3559, 1000.000000000000114 ) ;
#11881=EDGE_CURVE ( 'NONE', #3359, #1805, #12122, .T. ) ;
#11882=EDGE_CURVE ( 'NONE', #1013, #6387, #11122, .T. ) ;
#11886=CIRCLE ( 'NONE', #12391, 6.000000000000005329 ) ;
#11889=DIRECTION ( 'NONE',  ( 1.000000000000000000, 0.000000000000000000, 0.000000000000000000 ) ) ;
#11898=AXIS2_PLACEMENT_3D ( 'NONE', #9805, #2660, #14572 ) ;
#11901=CIRCLE ( 'NONE', #7250, 2.999999999999988898 ) ;
#11928=CARTESIAN_POINT ( 'NONE',  ( 93.63799900313688340, -2.337932895214617890, 2.999999999999999112 ) ) ;
#11971=CIRCLE ( 'NONE', #4887, 5.999999999999999112 ) ;
#11981=CARTESIAN_POINT ( 'NONE',  ( 93.34550147531103903, 3.654933296868752457, 6.000000000000000000 ) ) ;
#12001=CYLINDRICAL_SURFACE ( 'NONE', #7591, 4.000000000000000000 ) ;
#12020=DIRECTION ( 'NONE',  ( 0.000000000000000000, 0.000000000000000000, 1.000000000000000000 ) ) ;
#12023=CARTESIAN_POINT ( 'NONE',  ( 101.6227766016837819, 5.204170427930421283E-15, 6.000000000000005329 ) ) ;
#12037=VERTEX_POINT ( 'NONE', #5534 ) ;
#12056=DIRECTION ( 'NONE',  ( 1.000000000000000000, 0.000000000000000000, 0.000000000000000000 ) ) ;
#12092=PLANE ( 'NONE',  #10924 ) ;
#12107=FACE_OUTER_BOUND ( 'NONE', #10669, .T. ) ;
#12119=CIRCLE ( 'NONE', #5517, 6.000000000000000000 ) ;
#12122=LINE ( 'NONE', #6374, #5072 ) ;
#12142=ORIENTED_EDGE ( 'NONE', *, *, #6158, .F. ) ;
#12148=CYLINDRICAL_SURFACE ( 'NONE', #14630, 4.999999999999997335 ) ;
#12149=CIRCLE ( 'NONE', #9457, 4.000000000000003553 ) ;
#12157=CARTESIAN_POINT ( 'NONE',  ( 93.63799900313688340, -2.337932895214617890, 2.999999999999999112 ) ) ;
#12158=ORIENTED_EDGE ( 'NONE', *, *, #344, .F. ) ;
#12192=CYLINDRICAL_SURFACE ( 'NONE', #15168, 4.000000000000000000 ) ;
#12240=DIRECTION ( 'NONE',  ( -0.000000000000000000, -0.000000000000000000, -1.000000000000000000 ) ) ;
#12246=EDGE_CURVE ( 'NONE', #12877, #1013, #15138, .T. ) ;
#12255=( NAMED_UNIT ( * ) PLANE_ANGLE_UNIT ( ) SI_UNIT ( $, .RADIAN. ) );
#12280=DIRECTION ( 'NONE',  ( -0.000000000000000000, -0.000000000000000000, -1.000000000000000000 ) ) ;
#12283=DIRECTION ( 'NONE',  ( -1.000000000000000000, 0.000000000000000000, 0.000000000000000000 ) ) ;
#12299=CARTESIAN_POINT ( 'NONE',  ( 72.68384697807672978, 11.35494834827056110, 6.000000000000000000 ) ) ;
#12306=DIRECTION ( 'NONE',  ( -1.000000000000000000, 0.000000000000000000, 0.000000000000000000 ) ) ;
#12316=VERTEX_POINT ( 'NONE', #10134 ) ;
#12326=CARTESIAN_POINT ( 'NONE',  ( 0.000000000000000000, 0.000000000000000000, 6.000000000000000000 ) ) ;
#12328=EDGE_CURVE ( 'NONE', #7552, #3308, #7768, .T. ) ;
#12330=PLANE ( 'NONE',  #15114 ) ;
#12332=ORIENTED_EDGE ( 'NONE', *, *, #5705, .T. ) ;
#12355=DIRECTION ( 'NONE',  ( 0.000000000000000000, 0.000000000000000000, 1.000000000000000000 ) ) ;
#12366=LINE ( 'NONE', #7847, #3260 ) ;
#12368=DIRECTION ( 'NONE',  ( 1.000000000000000000, 0.000000000000000000, 0.000000000000000000 ) ) ;
#12370=AXIS2_PLACEMENT_3D ( 'NONE', #13455, #12457, #1704 ) ;
#12371=DIRECTION ( 'NONE',  ( -1.000000000000000000, 0.000000000000000000, 0.000000000000000000 ) ) ;
#12377=ORIENTED_EDGE ( 'NONE', *, *, #1603, .T. ) ;
#12380=ADVANCED_FACE ( 'NONE', ( #6524 ), #11206, .F. ) ;
#12391=AXIS2_PLACEMENT_3D ( 'NONE', #11640, #10726, #4901 ) ;
#12392=AXIS2_PLACEMENT_3D ( 'NONE', #10243, #11538, #14859 ) ;
#12402=CIRCLE ( 'NONE', #11898, 9.999999999999994671 ) ;
#12425=DIRECTION ( 'NONE',  ( 0.4571871344001384174, 0.8893705212896307888, 0.000000000000000000 ) ) ;
#12445=DIRECTION ( 'NONE',  ( -0.000000000000000000, -0.000000000000000000, 1.000000000000000000 ) ) ;
#12457=DIRECTION ( 'NONE',  ( -0.000000000000000000, -0.000000000000000000, -1.000000000000000000 ) ) ;
#12465=EDGE_CURVE ( 'NONE', #677, #11238, #12659, .T. ) ;
#12467=VECTOR ( 'NONE', #3351, 1000.000000000000000 ) ;
#12481=EDGE_LOOP ( 'NONE', ( #13258, #13002, #870, #5685 ) ) ;
#12482=CARTESIAN_POINT ( 'NONE',  ( 1.666666666666673624, 0.000000000000000000, 3.000000000000002665 ) ) ;
#12490=EDGE_CURVE ( 'NONE', #11633, #11133, #9290, .T. ) ;
#12506=CIRCLE ( 'NONE', #2701, 4.000000000000003553 ) ;
#12525=FACE_OUTER_BOUND ( 'NONE', #7084, .T. ) ;
#12549=CARTESIAN_POINT ( 'NONE',  ( 98.48580539929344013, 0.9022481406819604643, 6.000000000000000000 ) ) ;
#12551=ORIENTED_EDGE ( 'NONE', *, *, #6906, .T. ) ;
#12552=ORIENTED_EDGE ( 'NONE', *, *, #15030, .F. ) ;
#12558=CARTESIAN_POINT ( 'NONE',  ( 86.17559721729969624, 12.01344854909570259, 6.000000000000000000 ) ) ;
#12569=CARTESIAN_POINT ( 'NONE',  ( 85.79342132543153809, 17.83186255874426962, 2.999999999999999112 ) ) ;
#12570=DIRECTION ( 'NONE',  ( -0.5416238976136773520, 0.8406209333187990573, 0.000000000000000000 ) ) ;
#12603=VERTEX_POINT ( 'NONE', #13395 ) ;
#12612=LINE ( 'NONE', #5566, #1675 ) ;
#12629=DIRECTION ( 'NONE',  ( -1.000000000000000000, 0.000000000000000000, 0.000000000000000000 ) ) ;
#12638=AXIS2_PLACEMENT_3D ( 'NONE', #12697, #12838, #10554 ) ;
#12639=ORIENTED_EDGE ( 'NONE', *, *, #6906, .F. ) ;
#12641=FACE_OUTER_BOUND ( 'NONE', #9564, .T. ) ;
#12649=CARTESIAN_POINT ( 'NONE',  ( 14.40394475573011945, -10.79473832354794460, 5.500000000000001776 ) ) ;
#12651=ADVANCED_FACE ( 'NONE', ( #14790 ), #7569, .F. ) ;
#12652=EDGE_CURVE ( 'NONE', #12037, #12877, #4595, .T. ) ;
#12659=CIRCLE ( 'NONE', #11444, 3.000000000000002665 ) ;
#12670=AXIS2_PLACEMENT_3D ( 'NONE', #51, #8363, #13042 ) ;
#12675=VERTEX_POINT ( 'NONE', #11471 ) ;
#12679=ORIENTED_EDGE ( 'NONE', *, *, #7030, .T. ) ;
#12695=CIRCLE ( 'NONE', #8008, 4.999999999999997335 ) ;
#12697=CARTESIAN_POINT ( 'NONE',  ( 0.000000000000000000, 0.000000000000000000, 6.000000000000000000 ) ) ;
#12700=VERTEX_POINT ( 'NONE', #5793 ) ;
#12724=ORIENTED_EDGE ( 'NONE', *, *, #211, .T. ) ;
#12726=LINE ( 'NONE', #2356, #1524 ) ;
#12731=EDGE_CURVE ( 'NONE', #14436, #2991, #4075, .T. ) ;
#12745=LINE ( 'NONE', #6913, #1719 ) ;
#12765=ORIENTED_EDGE ( 'NONE', *, *, #6777, .T. ) ;
#12768=CARTESIAN_POINT ( 'NONE',  ( 84.00000000000000000, 0.000000000000000000, 6.000000000000000000 ) ) ;
#12769=VERTEX_POINT ( 'NONE', #3474 ) ;
#12780=DIRECTION ( 'NONE',  ( 0.000000000000000000, 0.000000000000000000, 1.000000000000000000 ) ) ;
#12795=CARTESIAN_POINT ( 'NONE',  ( 111.6227766016837961, 7.610970684806392799E-15, 3.000000000000002665 ) ) ;
#12802=DIRECTION ( 'NONE',  ( 0.000000000000000000, 0.000000000000000000, 1.000000000000000000 ) ) ;
#12806=CARTESIAN_POINT ( 'NONE',  ( 56.98919079003883326, 3.953582723775848962, 6.000000000000000000 ) ) ;
#12824=ORIENTED_EDGE ( 'NONE', *, *, #1732, .F. ) ;
#12825=DIRECTION ( 'NONE',  ( 0.000000000000000000, 0.000000000000000000, -1.000000000000000000 ) ) ;
#12832=LINE ( 'NONE', #11765, #14405 ) ;
#12838=DIRECTION ( 'NONE',  ( 0.000000000000000000, 0.000000000000000000, 1.000000000000000000 ) ) ;
#12844=FACE_OUTER_BOUND ( 'NONE', #6795, .T. ) ;
#12877=VERTEX_POINT ( 'NONE', #1174 ) ;
#12890=EDGE_CURVE ( 'NONE', #5429, #13724, #3810, .T. ) ;
#12896=CARTESIAN_POINT ( 'NONE',  ( 0.000000000000000000, 0.000000000000000000, 3.000000000000000000 ) ) ;
#12899=PLANE ( 'NONE',  #4036 ) ;
#12917=PRODUCT_DEFINITION ( 'UNKNOWN', '', #4021, #7630 ) ;
#12929=FACE_OUTER_BOUND ( 'NONE', #11144, .T. ) ;
#12930=CARTESIAN_POINT ( 'NONE',  ( 1.666666666666673624, 0.000000000000000000, 6.000000000000000000 ) ) ;
#12934=ORIENTED_EDGE ( 'NONE', *, *, #15017, .T. ) ;
#12952=EDGE_CURVE ( 'NONE', #5949, #13989, #9960, .T. ) ;
#12969=EDGE_LOOP ( 'NONE', ( #12551, #4688, #2877, #1669, #8805 ) ) ;
#12990=DIRECTION ( 'NONE',  ( 1.000000000000000000, 0.000000000000000000, 0.000000000000000000 ) ) ;
#13002=ORIENTED_EDGE ( 'NONE', *, *, #2621, .F. ) ;
#13013=APPLICATION_CONTEXT ( 'automotive_design' ) ;
#13041=AXIS2_PLACEMENT_3D ( 'NONE', #12649, #2133, #976 ) ;
#13042=DIRECTION ( 'NONE',  ( 1.000000000000000000, 0.000000000000000000, 0.000000000000000000 ) ) ;
#13056=CIRCLE ( 'NONE', #9878, 4.000000000000000000 ) ;
#13079=CARTESIAN_POINT ( 'NONE',  ( 86.17559721729969624, 12.01344854909570259, 2.999999999999999112 ) ) ;
#13086=CIRCLE ( 'NONE', #10655, 4.999999999999997335 ) ;
#13090=PLANE ( 'NONE',  #6596 ) ;
#13096=ORIENTED_EDGE ( 'NONE', *, *, #15017, .F. ) ;
#13105=CARTESIAN_POINT ( 'NONE',  ( 61.98919079003883326, 3.953582723775848962, 2.999999999999999112 ) ) ;
#13110=EDGE_LOOP ( 'NONE', ( #10664, #3684, #8717, #5087 ) ) ;
#13136=CARTESIAN_POINT ( 'NONE',  ( 14.40394475573011945, -10.79473832354794460, 3.000000000000000000 ) ) ;
#13169=ORIENTED_EDGE ( 'NONE', *, *, #1571, .T. ) ;
#13171=CARTESIAN_POINT ( 'NONE',  ( 8.961831343790189308, 9.104486995144791095, -131.1575142076926852 ) ) ;
#13184=CARTESIAN_POINT ( 'NONE',  ( 67.23404255319145761, 28.93147646537026318, 6.000000000000000000 ) ) ;
#13200=VERTEX_POINT ( 'NONE', #10313 ) ;
#13209=ORIENTED_EDGE ( 'NONE', *, *, #12731, .F. ) ;
#13226=VECTOR ( 'NONE', #3964, 1000.000000000000000 ) ;
#13232=CIRCLE ( 'NONE', #2191, 5.999999999999999112 ) ;
#13241=DIRECTION ( 'NONE',  ( -0.8893705212896292345, 0.4571871344001417481, 0.000000000000000000 ) ) ;
#13244=VERTEX_POINT ( 'NONE', #6150 ) ;
#13252=DIRECTION ( 'NONE',  ( -0.000000000000000000, -0.000000000000000000, 1.000000000000000000 ) ) ;
#13255=CARTESIAN_POINT ( 'NONE',  ( 56.98919079003883326, 3.953582723775848962, 2.999999999999999112 ) ) ;
#13256=FACE_BOUND ( 'NONE', #1075, .T. ) ;
#13258=ORIENTED_EDGE ( 'NONE', *, *, #9364, .F. ) ;
#13259=CARTESIAN_POINT ( 'NONE',  ( 91.46153288930040048, 16.46030115554384565, 6.000000000000000000 ) ) ;
#13288=ADVANCED_FACE ( 'NONE', ( #13997, #3529, #4936, #8218, #11675, #8299, #3463, #2536 ), #14225, .F. ) ;
#13295=ADVANCED_FACE ( 'NONE', ( #1300, #10682 ), #1161, .T. ) ;
#13311=EDGE_CURVE ( 'NONE', #5009, #10601, #7300, .T. ) ;
#13324=ADVANCED_FACE ( 'NONE', ( #3610 ), #1236, .T. ) ;
#13326=CARTESIAN_POINT ( 'NONE',  ( 93.34550147531103903, 3.654933296868752457, 2.999999999999999112 ) ) ;
#13333=EDGE_LOOP ( 'NONE', ( #481, #10894, #2467, #7325 ) ) ;
#13335=ADVANCED_FACE ( 'NONE', ( #8749 ), #9902, .F. ) ;
#13348=ORIENTED_EDGE ( 'NONE', *, *, #3697, .F. ) ;
#13374=CIRCLE ( 'NONE', #614, 20.00000000000000000 ) ;
#13395=CARTESIAN_POINT ( 'NONE',  ( 74.00000000000000000, 0.000000000000000000, 5.500000000000000000 ) ) ;
#13406=FACE_BOUND ( 'NONE', #3956, .T. ) ;
#13408=DIRECTION ( 'NONE',  ( -0.000000000000000000, -0.000000000000000000, 1.000000000000000000 ) ) ;
#13410=EDGE_LOOP ( 'NONE', ( #7612, #8497, #14432, #4209 ) ) ;
#13423=CARTESIAN_POINT ( 'NONE',  ( 33.82574562093736859, -6.697933970950280091, 2.999999999999999112 ) ) ;
#13425=SHAPE_DEFINITION_REPRESENTATION ( #7269, #2588 ) ;
#13433=CYLINDRICAL_SURFACE ( 'NONE', #708, 4.000000000000000000 ) ;
#13448=DIRECTION ( 'NONE',  ( -0.9728364810787194505, -0.2314933715733012987, 0.000000000000000000 ) ) ;
#13453=CIRCLE ( 'NONE', #4866, 3.000000000000002665 ) ;
#13454=VECTOR ( 'NONE', #4710, 1000.000000000000000 ) ;
#13455=CARTESIAN_POINT ( 'NONE',  ( 101.6227766016837819, 5.204170427930421283E-15, 3.000000000000002665 ) ) ;
#13480=ADVANCED_FACE ( 'NONE', ( #11583 ), #4229, .F. ) ;
#13514=DIRECTION ( 'NONE',  ( 0.000000000000000000, 0.000000000000000000, 1.000000000000000000 ) ) ;
#13532=DIRECTION ( 'NONE',  ( -0.000000000000000000, -0.000000000000000000, 1.000000000000000000 ) ) ;
#13546=CARTESIAN_POINT ( 'NONE',  ( 4.000000000000000000, 4.898587196589412829E-16, 6.000000000000000000 ) ) ;
#13554=ORIENTED_EDGE ( 'NONE', *, *, #12465, .T. ) ;
#13562=DIRECTION ( 'NONE',  ( -0.9728364810787194505, -0.2314933715733012987, 0.000000000000000000 ) ) ;
#13566=DIRECTION ( 'NONE',  ( 0.000000000000000000, 0.000000000000000000, -1.000000000000000000 ) ) ;
#13599=ORIENTED_EDGE ( 'NONE', *, *, #6293, .T. ) ;
#13615=ADVANCED_FACE ( 'NONE', ( #10524 ), #10591, .F. ) ;
#13617=CARTESIAN_POINT ( 'NONE',  ( 69.97572749000833880, 15.55805301486455683, 2.999999999999999112 ) ) ;
#13644=( NAMED_UNIT ( * ) PLANE_ANGLE_UNIT ( ) SI_UNIT ( $, .RADIAN. ) );
#13652=LINE ( 'NONE', #7822, #9931 ) ;
#13658=VERTEX_POINT ( 'NONE', #13978 ) ;
#13664=ORIENTED_EDGE ( 'NONE', *, *, #10110, .T. ) ;
#13689=AXIS2_PLACEMENT_3D ( 'NONE', #13326, #6120, #9643 ) ;
#13697=CARTESIAN_POINT ( 'NONE',  ( 72.68384697807672978, 11.35494834827056110, 6.000000000000000000 ) ) ;
#13703=DIRECTION ( 'NONE',  ( 0.000000000000000000, 0.000000000000000000, 1.000000000000000000 ) ) ;
#13705=DIRECTION ( 'NONE',  ( 0.000000000000000000, 0.000000000000000000, 1.000000000000000000 ) ) ;
#13718=SURFACE_STYLE_USAGE ( .BOTH. , #4426 ) ;
#13719=CARTESIAN_POINT ( 'NONE',  ( 75.20570977803312473, 12.97982004111159959, 2.999999999999999112 ) ) ;
#13724=VERTEX_POINT ( 'NONE', #9586 ) ;
#13731=VERTEX_POINT ( 'NONE', #11040 ) ;
#13743=CIRCLE ( 'NONE', #6638, 2.999999999999988898 ) ;
#13747=DIRECTION ( 'NONE',  ( 1.000000000000000000, 0.000000000000000000, 0.000000000000000000 ) ) ;
#13755=LINE ( 'NONE', #6759, #8206 ) ;
#13756=CIRCLE ( 'NONE', #3208, 4.000000000000000000 ) ;
#13765=EDGE_LOOP ( 'NONE', ( #14486, #5848, #8523, #10556 ) ) ;
#13776=DIRECTION ( 'NONE',  ( -0.000000000000000000, -0.000000000000000000, -1.000000000000000000 ) ) ;
#13810=FACE_BOUND ( 'NONE', #7494, .T. ) ;
#13834=ORIENTED_EDGE ( 'NONE', *, *, #1769, .T. ) ;
#13849=CIRCLE ( 'NONE', #5027, 31.62277660168379256 ) ;
#13859=EDGE_LOOP ( 'NONE', ( #12552, #2062, #7601, #5890 ) ) ;
#13886=EDGE_CURVE ( 'NONE', #6954, #3308, #4507, .T. ) ;
#13889=EDGE_LOOP ( 'NONE', ( #5168, #5927, #4854, #7305 ) ) ;
#13943=CARTESIAN_POINT ( 'NONE',  ( 19.25177984293773648, 7.759396820770405157, 3.000000000000002665 ) ) ;
#13947=CARTESIAN_POINT ( 'NONE',  ( 93.63799900313688340, -2.337932895214617890, 2.999999999999999112 ) ) ;
#13953=PLANE ( 'NONE',  #9984 ) ;
#13978=CARTESIAN_POINT ( 'NONE',  ( 18.40394475573011945, -10.79473832354794460, 5.500000000000000000 ) ) ;
#13981=DIRECTION ( 'NONE',  ( -0.000000000000000000, -0.000000000000000000, 1.000000000000000000 ) ) ;
#13989=VERTEX_POINT ( 'NONE', #9343 ) ;
#13997=FACE_BOUND ( 'NONE', #3823, .T. ) ;
#13998=CARTESIAN_POINT ( 'NONE',  ( -5.999999999999999112, 0.000000000000000000, 5.500000000000000000 ) ) ;
#14001=CARTESIAN_POINT ( 'NONE',  ( 83.50748565343083385, 13.38500995229612478, 2.999999999999999112 ) ) ;
#14029=FACE_OUTER_BOUND ( 'NONE', #13889, .T. ) ;
#14036=DIRECTION ( 'NONE',  ( 0.000000000000000000, 0.000000000000000000, 1.000000000000000000 ) ) ;
#14039=EDGE_LOOP ( 'NONE', ( #15006, #9314, #3923, #1559 ) ) ;
#14058=VECTOR ( 'NONE', #4959, 1000.000000000000000 ) ;
#14061=VERTEX_POINT ( 'NONE', #250 ) ;
#14062=CARTESIAN_POINT ( 'NONE',  ( 72.68384697807672978, 11.35494834827056110, 2.999999999999999112 ) ) ;
#14065=ADVANCED_FACE ( 'NONE', ( #9868 ), #2568, .F. ) ;
#14072=CARTESIAN_POINT ( 'NONE',  ( 67.45386469005195806, 13.93318132202354676, 2.999999999999999112 ) ) ;
#14078=ADVANCED_FACE ( 'NONE', ( #7422 ), #2879, .F. ) ;
#14084=EDGE_CURVE ( 'NONE', #12769, #12877, #3961, .T. ) ;
#14092=VECTOR ( 'NONE', #13448, 999.9999999999998863 ) ;
#14095=CYLINDRICAL_SURFACE ( 'NONE', #4858, 6.000000000000000000 ) ;
#14108=ORIENTED_EDGE ( 'NONE', *, *, #5813, .T. ) ;
#14113=DIRECTION ( 'NONE',  ( 1.000000000000000000, 0.000000000000000000, 0.000000000000000000 ) ) ;
#14120=ORIENTED_EDGE ( 'NONE', *, *, #5790, .T. ) ;
#14128=ORIENTED_EDGE ( 'NONE', *, *, #2429, .T. ) ;
#14129=CARTESIAN_POINT ( 'NONE',  ( -9.999999999999998224, -1.390791565672605534, -131.1575142076926852 ) ) ;
#14155=ADVANCED_FACE ( 'NONE', ( #2086 ), #5782, .T. ) ;
#14191=DIRECTION ( 'NONE',  ( 1.000000000000000000, 0.000000000000000000, 0.000000000000000000 ) ) ;
#14204=DIRECTION ( 'NONE',  ( 0.9728364810787193395, 0.2314933715733012431, 0.000000000000000000 ) ) ;
#14212=CARTESIAN_POINT ( 'NONE',  ( -9.999999999999992895, -25.00000000000000000, 6.000000000000000000 ) ) ;
#14225=PLANE ( 'NONE',  #4349 ) ;
#14250=ORIENTED_EDGE ( 'NONE', *, *, #1570, .F. ) ;
#14262=DIRECTION ( 'NONE',  ( -0.000000000000000000, -0.000000000000000000, 1.000000000000000000 ) ) ;
#14264=CARTESIAN_POINT ( 'NONE',  ( 111.6227766016837961, 7.610970684806392799E-15, -131.1575142076926852 ) ) ;
#14289=VECTOR ( 'NONE', #413, 1000.000000000000000 ) ;
#14295=EDGE_LOOP ( 'NONE', ( #10958, #6922 ) ) ;
#14297=DIRECTION ( 'NONE',  ( 1.000000000000000000, 0.000000000000000000, 0.000000000000000000 ) ) ;
#14307=EDGE_CURVE ( 'NONE', #6387, #12769, #3622, .T. ) ;
#14315=ORIENTED_EDGE ( 'NONE', *, *, #7407, .T. ) ;
#14317=DIRECTION ( 'NONE',  ( -0.000000000000000000, -0.000000000000000000, 1.000000000000000000 ) ) ;
#14322=DIRECTION ( 'NONE',  ( 0.000000000000000000, 0.000000000000000000, -1.000000000000000000 ) ) ;
#14324=LINE ( 'NONE', #243, #6944 ) ;
#14332=FACE_OUTER_BOUND ( 'NONE', #10255, .T. ) ;
#14339=CIRCLE ( 'NONE', #12370, 9.999999999999994671 ) ;
#14345=CARTESIAN_POINT ( 'NONE',  ( 83.50748565343083385, 13.38500995229612478, 6.000000000000000000 ) ) ;
#14352=ORIENTED_EDGE ( 'NONE', *, *, #2621, .T. ) ;
#14353=VECTOR ( 'NONE', #12283, 1000.000000000000000 ) ;
#14367=CARTESIAN_POINT ( 'NONE',  ( 80.00000000000000000, 0.000000000000000000, 6.000000000000000000 ) ) ;
#14388=AXIS2_PLACEMENT_3D ( 'NONE', #5030, #9620, #5191 ) ;
#14405=VECTOR ( 'NONE', #224, 1000.000000000000000 ) ;
#14414=VERTEX_POINT ( 'NONE', #9904 ) ;
#14419=FACE_BOUND ( 'NONE', #1532, .T. ) ;
#14422=AXIS2_PLACEMENT_3D ( 'NONE', #8131, #8199, #2290 ) ;
#14432=ORIENTED_EDGE ( 'NONE', *, *, #779, .F. ) ;
#14436=VERTEX_POINT ( 'NONE', #3074 ) ;
#14446=VERTEX_POINT ( 'NONE', #7759 ) ;
#14450=CARTESIAN_POINT ( 'NONE',  ( 14.40394475573011945, -10.79473832354794460, 6.000000000000000000 ) ) ;
#14454=ORIENTED_EDGE ( 'NONE', *, *, #7016, .F. ) ;
#14461=VERTEX_POINT ( 'NONE', #5399 ) ;
#14462=DIRECTION ( 'NONE',  ( 0.000000000000000000, 0.000000000000000000, 1.000000000000000000 ) ) ;
#14471=CIRCLE ( 'NONE', #2190, 6.000000000000005329 ) ;
#14473=VECTOR ( 'NONE', #9642, 1000.000000000000000 ) ;
#14474=ORIENTED_EDGE ( 'NONE', *, *, #6198, .F. ) ;
#14486=ORIENTED_EDGE ( 'NONE', *, *, #12246, .F. ) ;
#14515=ADVANCED_FACE ( 'NONE', ( #12525 ), #3158, .T. ) ;
#14526=LINE ( 'NONE', #5163, #1589 ) ;
#14538=CARTESIAN_POINT ( 'NONE',  ( 80.00000000000000000, 0.000000000000000000, 5.500000000000005329 ) ) ;
#14553=FACE_OUTER_BOUND ( 'NONE', #11279, .T. ) ;
#14567=ORIENTED_EDGE ( 'NONE', *, *, #511, .F. ) ;
#14571=FILL_AREA_STYLE_COLOUR ( '', #6577 ) ;
#14572=DIRECTION ( 'NONE',  ( 1.000000000000000000, 0.000000000000000000, 0.000000000000000000 ) ) ;
#14575=DIRECTION ( 'NONE',  ( -0.9863939238321436376, -0.1643989873053573192, 0.000000000000000000 ) ) ;
#14578=CARTESIAN_POINT ( 'NONE',  ( 54.00962148274520302, 34.79915921274093193, 6.000000000000000000 ) ) ;
#14617=CARTESIAN_POINT ( 'NONE',  ( 14.40394475573011945, -10.79473832354794460, 3.000000000000000000 ) ) ;
#14630=AXIS2_PLACEMENT_3D ( 'NONE', #4013, #14317, #5114 ) ;
#14657=CIRCLE ( 'NONE', #1392, 11.66666666666667318 ) ;
#14661=ORIENTED_EDGE ( 'NONE', *, *, #1247, .T. ) ;
#14667=AXIS2_PLACEMENT_3D ( 'NONE', #14911, #12445, #7840 ) ;
#14672=CIRCLE ( 'NONE', #5112, 4.000000000000003553 ) ;
#14676=DIRECTION ( 'NONE',  ( -1.000000000000000000, 0.000000000000000000, 0.000000000000000000 ) ) ;
#14685=AXIS2_PLACEMENT_3D ( 'NONE', #6886, #6592, #12570 ) ;
#14696=ORIENTED_EDGE ( 'NONE', *, *, #1603, .F. ) ;
#14704=ORIENTED_EDGE ( 'NONE', *, *, #8071, .T. ) ;
#14752=CARTESIAN_POINT ( 'NONE',  ( 0.000000000000000000, 0.000000000000000000, 5.500000000000000000 ) ) ;
#14759=DIRECTION ( 'NONE',  ( -0.000000000000000000, -0.000000000000000000, 1.000000000000000000 ) ) ;
#14763=CARTESIAN_POINT ( 'NONE',  ( 101.4858053992934401, 0.9022481406819604643, 2.999999999999999112 ) ) ;
#14773=ORIENTED_EDGE ( 'NONE', *, *, #12490, .F. ) ;
#14790=FACE_OUTER_BOUND ( 'NONE', #8602, .T. ) ;
#14804=DIRECTION ( 'NONE',  ( -0.000000000000000000, -0.000000000000000000, 1.000000000000000000 ) ) ;
#14805=ADVANCED_FACE ( 'NONE', ( #12107 ), #12192, .F. ) ;
#14854=VECTOR ( 'NONE', #1059, 1000.000000000000000 ) ;
#14859=DIRECTION ( 'NONE',  ( -1.000000000000000000, 0.000000000000000000, 0.000000000000000000 ) ) ;
#14868=EDGE_LOOP ( 'NONE', ( #4827, #8634, #8284, #11537 ) ) ;
#14875=ORIENTED_EDGE ( 'NONE', *, *, #8159, .T. ) ;
#14903=VECTOR ( 'NONE', #4945, 1000.000000000000114 ) ;
#14911=CARTESIAN_POINT ( 'NONE',  ( 93.49175023922396122, 0.6585002008270834928, 2.999999999999999112 ) ) ;
#14935=EDGE_CURVE ( 'NONE', #5508, #7872, #2680, .T. ) ;
#14994=EDGE_LOOP ( 'NONE', ( #6789, #4015 ) ) ;
#15006=ORIENTED_EDGE ( 'NONE', *, *, #3350, .F. ) ;
#15012=CARTESIAN_POINT ( 'NONE',  ( 91.12964445316929130, 15.08873975234342701, 3.000000000000000000 ) ) ;
#15017=EDGE_CURVE ( 'NONE', #8579, #5309, #11273, .T. ) ;
#15023=ORIENTED_EDGE ( 'NONE', *, *, #9161, .F. ) ;
#15027=VERTEX_POINT ( 'NONE', #5597 ) ;
#15030=EDGE_CURVE ( 'NONE', #9599, #6485, #9195, .T. ) ;
#15031=LINE ( 'NONE', #4661, #11872 ) ;
#15042=DIRECTION ( 'NONE',  ( -0.000000000000000000, -0.000000000000000000, -1.000000000000000000 ) ) ;
#15059=VERTEX_POINT ( 'NONE', #5518 ) ;
#15063=CARTESIAN_POINT ( 'NONE',  ( 80.00000000000000000, 0.000000000000000000, 3.000000000000000000 ) ) ;
#15090=CIRCLE ( 'NONE', #6250, 31.62277660168379256 ) ;
#15100=AXIS2_PLACEMENT_3D ( 'NONE', #3320, #11608, #4482 ) ;
#15106=FACE_OUTER_BOUND ( 'NONE', #10984, .T. ) ;
#15113=AXIS2_PLACEMENT_3D ( 'NONE', #4872, #5874, #12990 ) ;
#15114=AXIS2_PLACEMENT_3D ( 'NONE', #878, #11624, #2193 ) ;
#15124=DIRECTION ( 'NONE',  ( -0.000000000000000000, -0.000000000000000000, -1.000000000000000000 ) ) ;
#15133=CIRCLE ( 'NONE', #7279, 2.999999999999988898 ) ;
#15138=CIRCLE ( 'NONE', #10224, 10.00000000000000000 ) ;
#15168=AXIS2_PLACEMENT_3D ( 'NONE', #11190, #351, #501 ) ;
#15172=ADVANCED_BREP_SHAPE_REPRESENTATION ( '', ( #3822, #1376 ), #5367 ) ;
#15197=ORIENTED_EDGE ( 'NONE', *, *, #3329, .F. ) ;
#15212=CARTESIAN_POINT ( 'NONE',  ( 80.00000000000000000, 0.000000000000000000, 5.500000000000000000 ) ) ;
#15217=CIRCLE ( 'NONE', #1946, 2.999999999999975131 ) ;
#15252=COLOUR_RGB('Light Blue',0.38,0.62,0.78);
#15253=FILL_AREA_STYLE_COLOUR('',#15252);
#15254=FILL_AREA_STYLE('',(#15253));
#15255=SURFACE_STYLE_FILL_AREA(#15254);
#15256=SURFACE_SIDE_STYLE('',(#15255));
#15257=SURFACE_STYLE_USAGE(.BOTH.,#15256);
#15258=PRESENTATION_STYLE_ASSIGNMENT((#15257));
ENDSEC;
END-ISO-10303-21;
